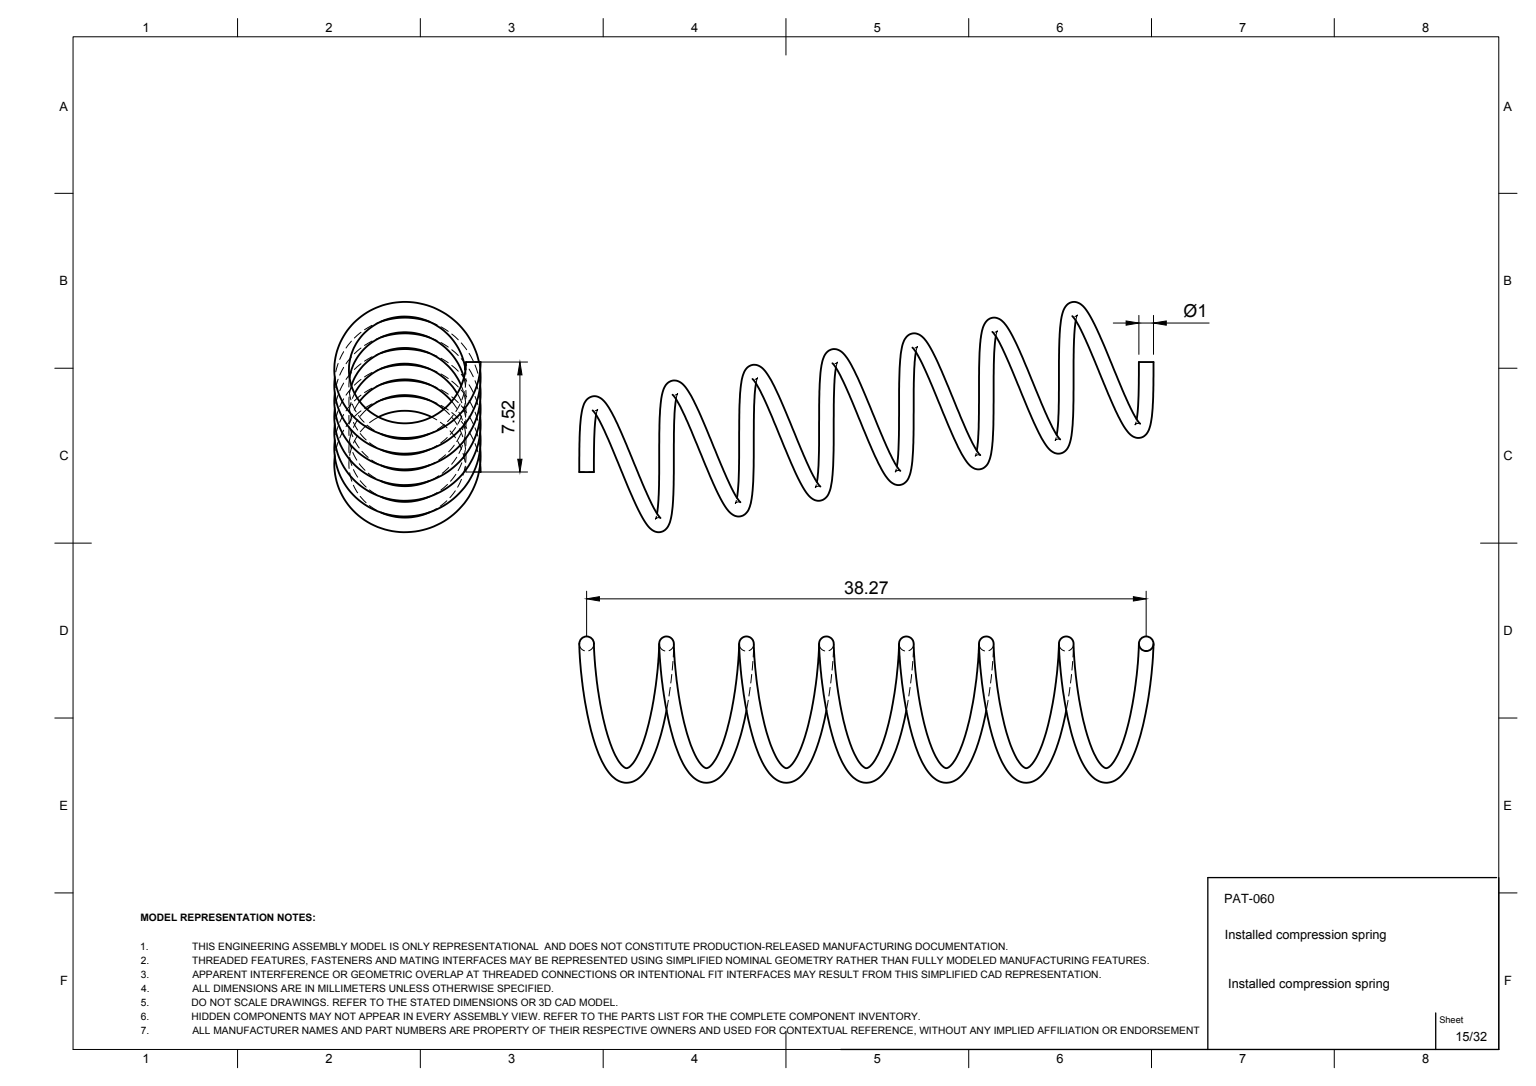
ISO-10303-21;
HEADER;
/* Generated by software containing ST-Developer
 * from STEP Tools, Inc. (www.steptools.com) 
 */

FILE_DESCRIPTION(
/* description */ ('Indexing fixture plate with plunger'),
/* implementation_level */ '2;1');

FILE_NAME(
/* name */ 'Installed compression spring.step',
/* time_stamp */ '2026-10-28T03:23:41-07:00',
/* author */ (''),
/* organization */ (''),
/* preprocessor_version */ 'ST-DEVELOPER v20.2',
/* originating_system */ 'Autodesk Translation Framework v15.17.0.0',
/* authorisation */ '');

FILE_SCHEMA (('AUTOMOTIVE_DESIGN { 1 0 10303 214 3 1 1 }'));
ENDSEC;

DATA;
#10=MECHANICAL_DESIGN_GEOMETRIC_PRESENTATION_REPRESENTATION('',(#327),#10020);
#233=B_SPLINE_SURFACE_WITH_KNOTS('',3,3,((#7454,#7455,#7456,#7457,#7458,
#7459,#7460,#7461,#7462,#7463,#7464,#7465,#7466,#7467,#7468,#7469,#7470,
#7471,#7472,#7473,#7474,#7475,#7476,#7477,#7478,#7479,#7480,#7481,#7482,
#7483,#7484,#7485,#7486,#7487,#7488,#7489,#7490,#7491,#7492,#7493,#7494,
#7495,#7496,#7497,#7498,#7499,#7500,#7501,#7502,#7503,#7504,#7505,#7506,
#7507,#7508,#7509,#7510,#7511,#7512,#7513,#7514,#7515,#7516,#7517,#7518,
#7519,#7520,#7521,#7522,#7523,#7524,#7525,#7526,#7527,#7528,#7529,#7530,
#7531,#7532,#7533,#7534,#7535,#7536,#7537,#7538,#7539,#7540,#7541,#7542,
#7543,#7544,#7545,#7546,#7547,#7548,#7549),(#7550,#7551,#7552,#7553,#7554,
#7555,#7556,#7557,#7558,#7559,#7560,#7561,#7562,#7563,#7564,#7565,#7566,
#7567,#7568,#7569,#7570,#7571,#7572,#7573,#7574,#7575,#7576,#7577,#7578,
#7579,#7580,#7581,#7582,#7583,#7584,#7585,#7586,#7587,#7588,#7589,#7590,
#7591,#7592,#7593,#7594,#7595,#7596,#7597,#7598,#7599,#7600,#7601,#7602,
#7603,#7604,#7605,#7606,#7607,#7608,#7609,#7610,#7611,#7612,#7613,#7614,
#7615,#7616,#7617,#7618,#7619,#7620,#7621,#7622,#7623,#7624,#7625,#7626,
#7627,#7628,#7629,#7630,#7631,#7632,#7633,#7634,#7635,#7636,#7637,#7638,
#7639,#7640,#7641,#7642,#7643,#7644,#7645),(#7646,#7647,#7648,#7649,#7650,
#7651,#7652,#7653,#7654,#7655,#7656,#7657,#7658,#7659,#7660,#7661,#7662,
#7663,#7664,#7665,#7666,#7667,#7668,#7669,#7670,#7671,#7672,#7673,#7674,
#7675,#7676,#7677,#7678,#7679,#7680,#7681,#7682,#7683,#7684,#7685,#7686,
#7687,#7688,#7689,#7690,#7691,#7692,#7693,#7694,#7695,#7696,#7697,#7698,
#7699,#7700,#7701,#7702,#7703,#7704,#7705,#7706,#7707,#7708,#7709,#7710,
#7711,#7712,#7713,#7714,#7715,#7716,#7717,#7718,#7719,#7720,#7721,#7722,
#7723,#7724,#7725,#7726,#7727,#7728,#7729,#7730,#7731,#7732,#7733,#7734,
#7735,#7736,#7737,#7738,#7739,#7740,#7741),(#7742,#7743,#7744,#7745,#7746,
#7747,#7748,#7749,#7750,#7751,#7752,#7753,#7754,#7755,#7756,#7757,#7758,
#7759,#7760,#7761,#7762,#7763,#7764,#7765,#7766,#7767,#7768,#7769,#7770,
#7771,#7772,#7773,#7774,#7775,#7776,#7777,#7778,#7779,#7780,#7781,#7782,
#7783,#7784,#7785,#7786,#7787,#7788,#7789,#7790,#7791,#7792,#7793,#7794,
#7795,#7796,#7797,#7798,#7799,#7800,#7801,#7802,#7803,#7804,#7805,#7806,
#7807,#7808,#7809,#7810,#7811,#7812,#7813,#7814,#7815,#7816,#7817,#7818,
#7819,#7820,#7821,#7822,#7823,#7824,#7825,#7826,#7827,#7828,#7829,#7830,
#7831,#7832,#7833,#7834,#7835,#7836,#7837),(#7838,#7839,#7840,#7841,#7842,
#7843,#7844,#7845,#7846,#7847,#7848,#7849,#7850,#7851,#7852,#7853,#7854,
#7855,#7856,#7857,#7858,#7859,#7860,#7861,#7862,#7863,#7864,#7865,#7866,
#7867,#7868,#7869,#7870,#7871,#7872,#7873,#7874,#7875,#7876,#7877,#7878,
#7879,#7880,#7881,#7882,#7883,#7884,#7885,#7886,#7887,#7888,#7889,#7890,
#7891,#7892,#7893,#7894,#7895,#7896,#7897,#7898,#7899,#7900,#7901,#7902,
#7903,#7904,#7905,#7906,#7907,#7908,#7909,#7910,#7911,#7912,#7913,#7914,
#7915,#7916,#7917,#7918,#7919,#7920,#7921,#7922,#7923,#7924,#7925,#7926,
#7927,#7928,#7929,#7930,#7931,#7932,#7933),(#7934,#7935,#7936,#7937,#7938,
#7939,#7940,#7941,#7942,#7943,#7944,#7945,#7946,#7947,#7948,#7949,#7950,
#7951,#7952,#7953,#7954,#7955,#7956,#7957,#7958,#7959,#7960,#7961,#7962,
#7963,#7964,#7965,#7966,#7967,#7968,#7969,#7970,#7971,#7972,#7973,#7974,
#7975,#7976,#7977,#7978,#7979,#7980,#7981,#7982,#7983,#7984,#7985,#7986,
#7987,#7988,#7989,#7990,#7991,#7992,#7993,#7994,#7995,#7996,#7997,#7998,
#7999,#8000,#8001,#8002,#8003,#8004,#8005,#8006,#8007,#8008,#8009,#8010,
#8011,#8012,#8013,#8014,#8015,#8016,#8017,#8018,#8019,#8020,#8021,#8022,
#8023,#8024,#8025,#8026,#8027,#8028,#8029),(#8030,#8031,#8032,#8033,#8034,
#8035,#8036,#8037,#8038,#8039,#8040,#8041,#8042,#8043,#8044,#8045,#8046,
#8047,#8048,#8049,#8050,#8051,#8052,#8053,#8054,#8055,#8056,#8057,#8058,
#8059,#8060,#8061,#8062,#8063,#8064,#8065,#8066,#8067,#8068,#8069,#8070,
#8071,#8072,#8073,#8074,#8075,#8076,#8077,#8078,#8079,#8080,#8081,#8082,
#8083,#8084,#8085,#8086,#8087,#8088,#8089,#8090,#8091,#8092,#8093,#8094,
#8095,#8096,#8097,#8098,#8099,#8100,#8101,#8102,#8103,#8104,#8105,#8106,
#8107,#8108,#8109,#8110,#8111,#8112,#8113,#8114,#8115,#8116,#8117,#8118,
#8119,#8120,#8121,#8122,#8123,#8124,#8125),(#8126,#8127,#8128,#8129,#8130,
#8131,#8132,#8133,#8134,#8135,#8136,#8137,#8138,#8139,#8140,#8141,#8142,
#8143,#8144,#8145,#8146,#8147,#8148,#8149,#8150,#8151,#8152,#8153,#8154,
#8155,#8156,#8157,#8158,#8159,#8160,#8161,#8162,#8163,#8164,#8165,#8166,
#8167,#8168,#8169,#8170,#8171,#8172,#8173,#8174,#8175,#8176,#8177,#8178,
#8179,#8180,#8181,#8182,#8183,#8184,#8185,#8186,#8187,#8188,#8189,#8190,
#8191,#8192,#8193,#8194,#8195,#8196,#8197,#8198,#8199,#8200,#8201,#8202,
#8203,#8204,#8205,#8206,#8207,#8208,#8209,#8210,#8211,#8212,#8213,#8214,
#8215,#8216,#8217,#8218,#8219,#8220,#8221),(#8222,#8223,#8224,#8225,#8226,
#8227,#8228,#8229,#8230,#8231,#8232,#8233,#8234,#8235,#8236,#8237,#8238,
#8239,#8240,#8241,#8242,#8243,#8244,#8245,#8246,#8247,#8248,#8249,#8250,
#8251,#8252,#8253,#8254,#8255,#8256,#8257,#8258,#8259,#8260,#8261,#8262,
#8263,#8264,#8265,#8266,#8267,#8268,#8269,#8270,#8271,#8272,#8273,#8274,
#8275,#8276,#8277,#8278,#8279,#8280,#8281,#8282,#8283,#8284,#8285,#8286,
#8287,#8288,#8289,#8290,#8291,#8292,#8293,#8294,#8295,#8296,#8297,#8298,
#8299,#8300,#8301,#8302,#8303,#8304,#8305,#8306,#8307,#8308,#8309,#8310,
#8311,#8312,#8313,#8314,#8315,#8316,#8317),(#8318,#8319,#8320,#8321,#8322,
#8323,#8324,#8325,#8326,#8327,#8328,#8329,#8330,#8331,#8332,#8333,#8334,
#8335,#8336,#8337,#8338,#8339,#8340,#8341,#8342,#8343,#8344,#8345,#8346,
#8347,#8348,#8349,#8350,#8351,#8352,#8353,#8354,#8355,#8356,#8357,#8358,
#8359,#8360,#8361,#8362,#8363,#8364,#8365,#8366,#8367,#8368,#8369,#8370,
#8371,#8372,#8373,#8374,#8375,#8376,#8377,#8378,#8379,#8380,#8381,#8382,
#8383,#8384,#8385,#8386,#8387,#8388,#8389,#8390,#8391,#8392,#8393,#8394,
#8395,#8396,#8397,#8398,#8399,#8400,#8401,#8402,#8403,#8404,#8405,#8406,
#8407,#8408,#8409,#8410,#8411,#8412,#8413)),.UNSPECIFIED.,.T.,.F.,.F.,(4,
1,1,1,1,1,1,4),(4,1,1,1,1,1,1,1,1,1,1,1,1,1,1,1,1,1,1,1,1,1,1,1,1,1,1,1,
1,1,1,1,1,1,1,1,1,1,1,1,1,1,1,1,1,1,1,1,1,1,1,1,1,1,1,1,1,1,1,1,1,1,1,1,
1,1,1,1,1,1,1,1,1,1,1,1,1,1,1,1,1,1,1,1,1,1,1,1,1,1,1,1,1,4),(-3.14159265358979,
-2.24399475256414,-1.34639685153848,-0.448798950512828,0.448798950512828,
1.34639685153848,2.24399475256414,3.14159265358979),(0.,0.00892857142857143,
0.0178571428571429,0.0267857142857143,0.0357142857142857,0.0446428571428571,
0.0535714285714286,0.0625,0.0714285714285714,0.0803571428571428,0.0892857142857143,
0.107142857142857,0.125,0.133928571428571,0.142857142857143,0.158730158730159,
0.174603174603175,0.19047619047619,0.202380952380952,0.214285714285714,
0.226190476190476,0.238095238095238,0.25,0.261904761904762,0.273809523809524,
0.285714285714286,0.297619047619048,0.30952380952381,0.321428571428571,
0.333333333333333,0.345238095238095,0.357142857142857,0.369047619047619,
0.375,0.380952380952381,0.392857142857143,0.404761904761905,0.416666666666667,
0.428571428571429,0.4375,0.446428571428571,0.455357142857143,0.464285714285714,
0.476190476190476,0.488095238095238,0.5,0.508928571428571,0.517857142857143,
0.535714285714286,0.553571428571429,0.571428571428571,0.580357142857143,
0.589285714285714,0.598214285714286,0.607142857142857,0.616071428571429,
0.625,0.633928571428571,0.642857142857143,0.654761904761905,0.666666666666667,
0.678571428571428,0.6875,0.696428571428571,0.705357142857143,0.714285714285714,
0.726190476190476,0.738095238095238,0.75,0.761904761904762,0.773809523809524,
0.785714285714286,0.797619047619047,0.809523809523809,0.821428571428571,
0.833333333333333,0.845238095238095,0.857142857142857,0.866071428571429,
0.875,0.883928571428571,0.892857142857143,0.901785714285714,0.910714285714286,
0.919642857142857,0.928571428571429,0.9375,0.946428571428571,0.955357142857143,
0.964285714285714,0.973214285714286,0.982142857142857,0.991071428571429,
1.),.UNSPECIFIED.);
#239=B_SPLINE_CURVE_WITH_KNOTS('',3,(#8417,#8418,#8419,#8420,#8421,#8422,
#8423,#8424,#8425,#8426,#8427,#8428,#8429,#8430,#8431,#8432,#8433,#8434,
#8435,#8436,#8437,#8438,#8439,#8440,#8441,#8442,#8443,#8444,#8445,#8446,
#8447,#8448,#8449,#8450,#8451,#8452,#8453,#8454,#8455,#8456,#8457,#8458,
#8459,#8460,#8461,#8462,#8463,#8464,#8465,#8466,#8467,#8468,#8469,#8470,
#8471,#8472,#8473,#8474,#8475,#8476,#8477,#8478,#8479,#8480,#8481,#8482,
#8483,#8484,#8485,#8486,#8487,#8488,#8489,#8490,#8491,#8492,#8493,#8494,
#8495,#8496,#8497,#8498,#8499,#8500,#8501,#8502,#8503,#8504,#8505,#8506,
#8507,#8508,#8509,#8510,#8511,#8512),.UNSPECIFIED.,.F.,.F.,(4,1,1,1,1,1,
1,1,1,1,1,1,1,1,1,1,1,1,1,1,1,1,1,1,1,1,1,1,1,1,1,1,1,1,1,1,1,1,1,1,1,1,
1,1,1,1,1,1,1,1,1,1,1,1,1,1,1,1,1,1,1,1,1,1,1,1,1,1,1,1,1,1,1,1,1,1,1,1,
1,1,1,1,1,1,1,1,1,1,1,1,1,1,1,4),(0.,0.00892857142857143,0.0178571428571429,
0.0267857142857143,0.0357142857142857,0.0446428571428571,0.0535714285714286,
0.0625,0.0714285714285714,0.0803571428571428,0.0892857142857143,0.107142857142857,
0.125,0.133928571428571,0.142857142857143,0.158730158730159,0.174603174603175,
0.19047619047619,0.202380952380952,0.214285714285714,0.226190476190476,
0.238095238095238,0.25,0.261904761904762,0.273809523809524,0.285714285714286,
0.297619047619048,0.30952380952381,0.321428571428571,0.333333333333333,
0.345238095238095,0.357142857142857,0.369047619047619,0.375,0.380952380952381,
0.392857142857143,0.404761904761905,0.416666666666667,0.428571428571429,
0.4375,0.446428571428571,0.455357142857143,0.464285714285714,0.476190476190476,
0.488095238095238,0.5,0.508928571428571,0.517857142857143,0.535714285714286,
0.553571428571429,0.571428571428571,0.580357142857143,0.589285714285714,
0.598214285714286,0.607142857142857,0.616071428571429,0.625,0.633928571428571,
0.642857142857143,0.654761904761905,0.666666666666667,0.678571428571428,
0.6875,0.696428571428571,0.705357142857143,0.714285714285714,0.726190476190476,
0.738095238095238,0.75,0.761904761904762,0.773809523809524,0.785714285714286,
0.797619047619047,0.809523809523809,0.821428571428571,0.833333333333333,
0.845238095238095,0.857142857142857,0.866071428571429,0.875,0.883928571428571,
0.892857142857143,0.901785714285714,0.910714285714286,0.919642857142857,
0.928571428571429,0.9375,0.946428571428571,0.955357142857143,0.964285714285714,
0.973214285714286,0.982142857142857,0.991071428571429,1.),.UNSPECIFIED.);
#273=SHAPE_REPRESENTATION_RELATIONSHIP('SRR','None',#10147,#300);
#300=ADVANCED_BREP_SHAPE_REPRESENTATION('',(#363),#10000);
#327=STYLED_ITEM('',(#10368),#363);
#363=MANIFOLD_SOLID_BREP('Body1',#4581);
#568=PLANE('',#5049);
#569=PLANE('',#5050);
#733=FACE_OUTER_BOUND('',#1060,.T.);
#734=FACE_OUTER_BOUND('',#1061,.T.);
#735=FACE_OUTER_BOUND('',#1062,.T.);
#1060=EDGE_LOOP('',(#3293,#3294,#3295,#3296));
#1061=EDGE_LOOP('',(#3297));
#1062=EDGE_LOOP('',(#3298));
#1896=CIRCLE('',#5047,0.05);
#1897=CIRCLE('',#5048,0.05);
#2212=VERTEX_POINT('',#8414);
#2213=VERTEX_POINT('',#8416);
#2626=EDGE_CURVE('',#2212,#2212,#1896,.T.);
#2627=EDGE_CURVE('',#2212,#2213,#239,.T.);
#2628=EDGE_CURVE('',#2213,#2213,#1897,.T.);
#3293=ORIENTED_EDGE('',*,*,#2626,.T.);
#3294=ORIENTED_EDGE('',*,*,#2627,.T.);
#3295=ORIENTED_EDGE('',*,*,#2628,.F.);
#3296=ORIENTED_EDGE('',*,*,#2627,.F.);
#3297=ORIENTED_EDGE('',*,*,#2628,.T.);
#3298=ORIENTED_EDGE('',*,*,#2626,.F.);
#4348=ADVANCED_FACE('',(#733),#233,.T.);
#4349=ADVANCED_FACE('',(#734),#568,.T.);
#4350=ADVANCED_FACE('',(#735),#569,.F.);
#4581=CLOSED_SHELL('',(#4348,#4349,#4350));
#5046=AXIS2_PLACEMENT_3D('',#7453,#5897,#5898);
#5047=AXIS2_PLACEMENT_3D('',#8415,#5899,#5900);
#5048=AXIS2_PLACEMENT_3D('',#8513,#5901,#5902);
#5049=AXIS2_PLACEMENT_3D('',#8514,#5903,#5904);
#5050=AXIS2_PLACEMENT_3D('',#8515,#5905,#5906);
#5897=DIRECTION('axis',(0.,0.,1.));
#5898=DIRECTION('refdir',(1.,0.,0.));
#5899=DIRECTION('center_axis',(-0.000132267085706657,0.981242764302753,
0.192776087751852));
#5900=DIRECTION('ref_axis',(2.59853443172113E-5,-0.192776086000499,0.981242773217255));
#5901=DIRECTION('center_axis',(0.000132265595059966,0.981242764048193,0.192776089048605));
#5902=DIRECTION('ref_axis',(-0.796598144949105,0.116638308439033,-0.593149981428075));
#5903=DIRECTION('center_axis',(0.000132265595059966,0.981242764048193,0.192776089048605));
#5904=DIRECTION('ref_axis',(-0.796598144949105,0.116638308439033,-0.593149981428075));
#5905=DIRECTION('center_axis',(-0.000132267085706657,0.981242764302753,
0.192776087751852));
#5906=DIRECTION('ref_axis',(2.59853443172113E-5,-0.192776086000499,0.981242773217256));
#7453=CARTESIAN_POINT('',(0.,0.,0.));
#7454=CARTESIAN_POINT('Ctrl Pts',(7.64999870073278,0.00963880430002493,
0.500937861339137));
#7455=CARTESIAN_POINT('Ctrl Pts',(7.64999072283273,0.0688240253405825,0.512565458280486));
#7456=CARTESIAN_POINT('Ctrl Pts',(7.62651906829351,0.186933280416436,0.535860737255745));
#7457=CARTESIAN_POINT('Ctrl Pts',(7.52538952050926,0.338721501716328,0.571111621876026));
#7458=CARTESIAN_POINT('Ctrl Pts',(7.37261016576107,0.440828782725881,0.606632113855559));
#7459=CARTESIAN_POINT('Ctrl Pts',(7.19098801918939,0.477160089388571,0.642432691908446));
#7460=CARTESIAN_POINT('Ctrl Pts',(7.00794887133667,0.440792445335284,0.678501299793522));
#7461=CARTESIAN_POINT('Ctrl Pts',(6.85151949944076,0.336499171833787,0.714833893830788));
#7462=CARTESIAN_POINT('Ctrl Pts',(6.74635289761356,0.179164878106423,0.751420068859459));
#7463=CARTESIAN_POINT('Ctrl Pts',(6.7088855037237,-0.00779582609077112,
0.78825059826266));
#7464=CARTESIAN_POINT('Ctrl Pts',(6.74651391108833,-0.195622387289353,0.825313313466632));
#7465=CARTESIAN_POINT('Ctrl Pts',(6.88851119015049,-0.410310488976418,0.875022999496246));
#7466=CARTESIAN_POINT('Ctrl Pts',(7.20522985356176,-0.542753193552164,0.937673401670968));
#7467=CARTESIAN_POINT('Ctrl Pts',(7.52560124560565,-0.410308950963103,1.00090311405878));
#7468=CARTESIAN_POINT('Ctrl Pts',(7.67086762315913,-0.190619832396083,1.0517623380234));
#7469=CARTESIAN_POINT('Ctrl Pts',(7.72038428103372,0.053554354178951,1.09994516441643));
#7470=CARTESIAN_POINT('Ctrl Pts',(7.61346157902179,0.349425527858921,1.15825605943124));
#7471=CARTESIAN_POINT('Ctrl Pts',(7.293147036645,0.533923363778534,1.22671892603372));
#7472=CARTESIAN_POINT('Ctrl Pts',(6.9598052915743,0.475238618295502,1.28954716027338));
#7473=CARTESIAN_POINT('Ctrl Pts',(6.74803078150055,0.262318163018047,1.34663189357301));
#7474=CARTESIAN_POINT('Ctrl Pts',(6.67830810206772,0.0023988076890563,1.3979329504908));
#7475=CARTESIAN_POINT('Ctrl Pts',(6.74786353789082,-0.257385664114871,1.44910892564238));
#7476=CARTESIAN_POINT('Ctrl Pts',(6.93745136291826,-0.446625861944449,1.50011118169226));
#7477=CARTESIAN_POINT('Ctrl Pts',(7.19511270617401,-0.515530236866011,1.55089291586215));
#7478=CARTESIAN_POINT('Ctrl Pts',(7.45136837615866,-0.446648689171563,1.60140954707133));
#7479=CARTESIAN_POINT('Ctrl Pts',(7.63768442718454,-0.260018056286165,1.65161922462518));
#7480=CARTESIAN_POINT('Ctrl Pts',(7.70523033687804,-0.0069714683683192,
1.70148323387221));
#7481=CARTESIAN_POINT('Ctrl Pts',(7.63769895751989,0.244003419049979,1.75096640161628));
#7482=CARTESIAN_POINT('Ctrl Pts',(7.45523859330254,0.426040600914326,1.80003745460796));
#7483=CARTESIAN_POINT('Ctrl Pts',(7.20843773134158,0.491855409637758,1.84866933496872));
#7484=CARTESIAN_POINT('Ctrl Pts',(6.96411419073211,0.426044527968114,1.89683949153479));
#7485=CARTESIAN_POINT('Ctrl Pts',(6.7872702247347,0.248717255937941,1.94453007704133));
#7486=CARTESIAN_POINT('Ctrl Pts',(6.72333142706999,0.00910740273079913,
1.99172820696913));
#7487=CARTESIAN_POINT('Ctrl Pts',(6.77669190792476,-0.188112629887261,2.03064296753181));
#7488=CARTESIAN_POINT('Ctrl Pts',(6.87311288530633,-0.313353108724919,2.06152326719269));
#7489=CARTESIAN_POINT('Ctrl Pts',(6.9977575234091,-0.409174440391491,2.0922362142172));
#7490=CARTESIAN_POINT('Ctrl Pts',(7.19095586866206,-0.460713817161615,2.13031448846159));
#7491=CARTESIAN_POINT('Ctrl Pts',(7.42021304552618,-0.399036009194613,2.17551521533059));
#7492=CARTESIAN_POINT('Ctrl Pts',(7.58607675038944,-0.232652998639623,2.22023530187249));
#7493=CARTESIAN_POINT('Ctrl Pts',(7.64084113722653,-0.0267711157317457,
2.2608041635776));
#7494=CARTESIAN_POINT('Ctrl Pts',(7.60365245023964,0.158696418911201,2.2973634945418));
#7495=CARTESIAN_POINT('Ctrl Pts',(7.50973838584388,0.299219822341778,2.33003006433835));
#7496=CARTESIAN_POINT('Ctrl Pts',(7.37007100234203,0.392281683236922,2.36247215334549));
#7497=CARTESIAN_POINT('Ctrl Pts',(7.18832364110351,0.428509871500047,2.39828479951764));
#7498=CARTESIAN_POINT('Ctrl Pts',(6.98993152312495,0.375130255900093,2.43739940337039));
#7499=CARTESIAN_POINT('Ctrl Pts',(6.83283942785452,0.217642962930976,2.47976008769737));
#7500=CARTESIAN_POINT('Ctrl Pts',(6.7805179762894,0.0217759129571612,2.51834494637949));
#7501=CARTESIAN_POINT('Ctrl Pts',(6.81611962546049,-0.155110783437508,2.55325894844757));
#7502=CARTESIAN_POINT('Ctrl Pts',(6.93559514558806,-0.335467183812974,2.59501419582854));
#7503=CARTESIAN_POINT('Ctrl Pts',(7.19838636703693,-0.444497554803198,2.64699296075227));
#7504=CARTESIAN_POINT('Ctrl Pts',(7.51396784981042,-0.313675439428632,2.70919005501935));
#7505=CARTESIAN_POINT('Ctrl Pts',(7.62212313812957,-0.0514208051434247,
2.76101600110827));
#7506=CARTESIAN_POINT('Ctrl Pts',(7.57941022831611,0.159498854704775,2.80255943176652));
#7507=CARTESIAN_POINT('Ctrl Pts',(7.49002790476542,0.293811387305209,2.83377939972915));
#7508=CARTESIAN_POINT('Ctrl Pts',(7.3552499441484,0.383795703607156,2.86508254302445));
#7509=CARTESIAN_POINT('Ctrl Pts',(7.19595280633545,0.41560735445773,2.89648910888395));
#7510=CARTESIAN_POINT('Ctrl Pts',(7.03593949389396,0.383792650446306,2.92801879141503));
#7511=CARTESIAN_POINT('Ctrl Pts',(6.89961651509014,0.292876470296345,2.95969053299985));
#7512=CARTESIAN_POINT('Ctrl Pts',(6.8081238548802,0.155952445855146,2.99152250722056));
#7513=CARTESIAN_POINT('Ctrl Pts',(6.7719951154116,-0.0244720795860329,3.02708849903104));
#7514=CARTESIAN_POINT('Ctrl Pts',(6.82508694038131,-0.224423780156864,3.0664872528009));
#7515=CARTESIAN_POINT('Ctrl Pts',(6.9861130399098,-0.385566648672682,3.1098474493302));
#7516=CARTESIAN_POINT('Ctrl Pts',(7.18949761386412,-0.440411898981026,3.14997109794484));
#7517=CARTESIAN_POINT('Ctrl Pts',(7.37626527013998,-0.403213775048244,3.18676673081186));
#7518=CARTESIAN_POINT('Ctrl Pts',(7.51993103796524,-0.30750405465344,3.2201390303787));
#7519=CARTESIAN_POINT('Ctrl Pts',(7.61665044076158,-0.16281791922389,3.25377599756719));
#7520=CARTESIAN_POINT('Ctrl Pts',(7.65498225700094,0.0283123086785322,3.29145196922942));
#7521=CARTESIAN_POINT('Ctrl Pts',(7.59852316170633,0.240631420079613,3.3332902111484));
#7522=CARTESIAN_POINT('Ctrl Pts',(7.42736589163809,0.412328652603764,3.37943210760514));
#7523=CARTESIAN_POINT('Ctrl Pts',(7.19081184831391,0.475941162716025,3.42607713455886));
#7524=CARTESIAN_POINT('Ctrl Pts',(6.95151342469985,0.412204069493947,3.47322302929114));
#7525=CARTESIAN_POINT('Ctrl Pts',(6.77437422620912,0.235528496642651,3.52086247665056));
#7526=CARTESIAN_POINT('Ctrl Pts',(6.70856719057301,-0.00853695568196444,
3.56898306053165));
#7527=CARTESIAN_POINT('Ctrl Pts',(6.77444746404088,-0.255049338492359,3.61756749823055));
#7528=CARTESIAN_POINT('Ctrl Pts',(6.9562898685306,-0.437346140614658,3.66659366870206));
#7529=CARTESIAN_POINT('Ctrl Pts',(7.20705837195632,-0.504822359013845,3.71603499825878));
#7530=CARTESIAN_POINT('Ctrl Pts',(7.45987118758895,-0.437340247483335,3.76586064283255));
#7531=CARTESIAN_POINT('Ctrl Pts',(7.64643847266503,-0.251145802482984,3.81603581337119));
#7532=CARTESIAN_POINT('Ctrl Pts',(7.70939130979041,-0.0164226811455054,
3.86231497498143));
#7533=CARTESIAN_POINT('Ctrl Pts',(7.66665300702434,0.198091300428752,3.90458351454994));
#7534=CARTESIAN_POINT('Ctrl Pts',(7.55703831361006,0.362363180751678,3.94275824199772));
#7535=CARTESIAN_POINT('Ctrl Pts',(7.39231161872226,0.472405147713809,3.98104671473859));
#7536=CARTESIAN_POINT('Ctrl Pts',(7.19757748614764,0.511253819560404,4.01942894411337));
#7537=CARTESIAN_POINT('Ctrl Pts',(7.00243742159468,0.472394913482402,4.05788442705078));
#7538=CARTESIAN_POINT('Ctrl Pts',(6.83675859423202,0.361776141956741,4.09639221672569));
#7539=CARTESIAN_POINT('Ctrl Pts',(6.72593678453896,0.195994806221917,4.13493108529455));
#7540=CARTESIAN_POINT('Ctrl Pts',(6.6870196897812,0.000372767277272366,
4.17347960299015));
#7541=CARTESIAN_POINT('Ctrl Pts',(6.72599808190112,-0.19515902350661,4.21201632288769));
#7542=CARTESIAN_POINT('Ctrl Pts',(6.83662574734572,-0.360840864201945,4.25051978478148));
#7543=CARTESIAN_POINT('Ctrl Pts',(7.00208504736442,-0.47127212461887,4.28896891774833));
#7544=CARTESIAN_POINT('Ctrl Pts',(7.19679737636779,-0.510060779189973,4.32734248506513));
#7545=CARTESIAN_POINT('Ctrl Pts',(7.39100313831524,-0.471299286801184,4.36562087591661));
#7546=CARTESIAN_POINT('Ctrl Pts',(7.5551719819179,-0.361667391724164,4.40378216412631));
#7547=CARTESIAN_POINT('Ctrl Pts',(7.66435033350436,-0.197951056928272,4.44181269280615));
#7548=CARTESIAN_POINT('Ctrl Pts',(7.68982126235038,-0.0699660743691742,
4.46705762798012));
#7549=CARTESIAN_POINT('Ctrl Pts',(7.68982990724746,-0.00583191542195246,
4.4796574990714));
#7550=CARTESIAN_POINT('Ctrl Pts',(7.6350387358516,0.00963678776443446,0.500937861339137));
#7551=CARTESIAN_POINT('Ctrl Pts',(7.63503101014841,0.0669510493656743,0.512197887426284));
#7552=CARTESIAN_POINT('Ctrl Pts',(7.61231574924475,0.1812935300152,0.5347473807854));
#7553=CARTESIAN_POINT('Ctrl Pts',(7.51437536109004,0.328330400226009,0.568888525111363));
#7554=CARTESIAN_POINT('Ctrl Pts',(7.36630661624771,0.427307066398246,0.603312533918598));
#7555=CARTESIAN_POINT('Ctrl Pts',(7.19013369937419,0.462570873330364,0.638036216400197));
#7556=CARTESIAN_POINT('Ctrl Pts',(7.01240713420346,0.42727728453773,0.673054009319043));
#7557=CARTESIAN_POINT('Ctrl Pts',(6.86033508130397,0.325921179563573,0.70836726659389));
#7558=CARTESIAN_POINT('Ctrl Pts',(6.7579611971146,0.172802978923407,0.74397206566071));
#7559=CARTESIAN_POINT('Ctrl Pts',(6.7214123199082,-0.00940771975300016,
0.779864408487187));
#7560=CARTESIAN_POINT('Ctrl Pts',(6.7581198571664,-0.192756797259193,0.816037450325855));
#7561=CARTESIAN_POINT('Ctrl Pts',(6.89690232809005,-0.402672103199899,0.86463407058812));
#7562=CARTESIAN_POINT('Ctrl Pts',(7.20725605051053,-0.532709504267443,0.926031233812609));
#7563=CARTESIAN_POINT('Ctrl Pts',(7.52258283785506,-0.402635707082477,0.988237247131344));
#7564=CARTESIAN_POINT('Ctrl Pts',(7.66601723416036,-0.185829339954806,1.0384238006937));
#7565=CARTESIAN_POINT('Ctrl Pts',(7.71503355357269,0.0556422780873975,1.08607199043942));
#7566=CARTESIAN_POINT('Ctrl Pts',(7.60918637088204,0.349162880547258,1.14388762640479));
#7567=CARTESIAN_POINT('Ctrl Pts',(7.2903515128854,0.533103613911741,1.21204744313397));
#7568=CARTESIAN_POINT('Ctrl Pts',(6.95707366748621,0.474656316327783,1.27485358832891));
#7569=CARTESIAN_POINT('Ctrl Pts',(6.74456178112433,0.261169820551568,1.33209897131474));
#7570=CARTESIAN_POINT('Ctrl Pts',(6.67433527221315,-0.000269397014741131,
1.38369681229794));
#7571=CARTESIAN_POINT('Ctrl Pts',(6.74440593081803,-0.262373809003338,1.43532105174058));
#7572=CARTESIAN_POINT('Ctrl Pts',(6.93612728066397,-0.453872081669123,1.48690459984704));
#7573=CARTESIAN_POINT('Ctrl Pts',(7.19745122001508,-0.523848922372219,1.53840681076736));
#7574=CARTESIAN_POINT('Ctrl Pts',(7.45805997886714,-0.453883269663763,1.58977025772498));
#7575=CARTESIAN_POINT('Ctrl Pts',(7.64803983262086,-0.263693101035238,1.64094678753314));
#7576=CARTESIAN_POINT('Ctrl Pts',(7.71711952609534,-0.00517849878257243,
1.69188667453881));
#7577=CARTESIAN_POINT('Ctrl Pts',(7.64804216604535,0.251791239903175,1.74254418096352));
#7578=CARTESIAN_POINT('Ctrl Pts',(7.46092188629594,0.438558185201571,1.79287579243366));
#7579=CARTESIAN_POINT('Ctrl Pts',(7.20735063505956,0.506228936588262,1.8428415890961));
#7580=CARTESIAN_POINT('Ctrl Pts',(6.95593925559357,0.438549903941295,1.89240539488024));
#7581=CARTESIAN_POINT('Ctrl Pts',(6.77373440484268,0.255889979988123,1.94153491121713));
#7582=CARTESIAN_POINT('Ctrl Pts',(6.70778531151454,0.00882356266419227,
1.99020293693628));
#7583=CARTESIAN_POINT('Ctrl Pts',(6.76283355713105,-0.194668074958629,2.0303550609426));
#7584=CARTESIAN_POINT('Ctrl Pts',(6.86234426891409,-0.323919294450078,2.06222522567205));
#7585=CARTESIAN_POINT('Ctrl Pts',(6.99099241075521,-0.4228168735756,2.09392553998431));
#7586=CARTESIAN_POINT('Ctrl Pts',(7.19040501251761,-0.476002229606067,2.1332315590035));
#7587=CARTESIAN_POINT('Ctrl Pts',(7.42694509743174,-0.412343436770496,2.17987197648186));
#7588=CARTESIAN_POINT('Ctrl Pts',(7.59795477669367,-0.24075224108209,2.22599099832676));
#7589=CARTESIAN_POINT('Ctrl Pts',(7.65432879696381,-0.0286540038200118,
2.26778999749925));
#7590=CARTESIAN_POINT('Ctrl Pts',(7.61604593360169,0.162166641626849,2.30540718503675));
#7591=CARTESIAN_POINT('Ctrl Pts',(7.51950918270181,0.306566623965249,2.33898210158965));
#7592=CARTESIAN_POINT('Ctrl Pts',(7.37615986978507,0.402052531958415,2.3722797613854));
#7593=CARTESIAN_POINT('Ctrl Pts',(7.18991757189564,0.439140491267482,2.40898011568004));
#7594=CARTESIAN_POINT('Ctrl Pts',(6.98704945595601,0.384483438050293,2.44898977868643));
#7595=CARTESIAN_POINT('Ctrl Pts',(6.82687936658702,0.223795186966439,2.49220010365028));
#7596=CARTESIAN_POINT('Ctrl Pts',(6.77374406457618,0.0245525470923147,2.53145813471135));
#7597=CARTESIAN_POINT('Ctrl Pts',(6.80989272676198,-0.154854651698435,2.56687895662991));
#7598=CARTESIAN_POINT('Ctrl Pts',(6.93084711889443,-0.337336060775077,2.60913936898076));
#7599=CARTESIAN_POINT('Ctrl Pts',(7.19586714485277,-0.446979863060233,2.66154817199395));
#7600=CARTESIAN_POINT('Ctrl Pts',(7.51214995264661,-0.315456586630328,2.72392487242511));
#7601=CARTESIAN_POINT('Ctrl Pts',(7.61973089828985,-0.0538169044635309,
2.77562308796219));
#7602=CARTESIAN_POINT('Ctrl Pts',(7.57725516276559,0.155639272831775,2.81688936140585));
#7603=CARTESIAN_POINT('Ctrl Pts',(7.48867898425771,0.288669487348,2.84782028505493));
#7604=CARTESIAN_POINT('Ctrl Pts',(7.35549434227958,0.377544841875494,2.8787535369846));
#7605=CARTESIAN_POINT('Ctrl Pts',(7.19848583194038,0.408858679622143,2.90971124099487));
#7606=CARTESIAN_POINT('Ctrl Pts',(7.0411630337891,0.37754703996107,2.94071683444724));
#7607=CARTESIAN_POINT('Ctrl Pts',(6.90744882895457,0.288327999365551,2.97179002108998));
#7608=CARTESIAN_POINT('Ctrl Pts',(6.8179071425464,0.154275853325778,3.00295604846018));
#7609=CARTESIAN_POINT('Ctrl Pts',(6.78264236297597,-0.0220015791954167,
3.03770458582966));
#7610=CARTESIAN_POINT('Ctrl Pts',(6.8344572243931,-0.216935347146573,3.07612357321105));
#7611=CARTESIAN_POINT('Ctrl Pts',(6.99115063676539,-0.373674687144112,3.11831302609281));
#7612=CARTESIAN_POINT('Ctrl Pts',(7.18868631032597,-0.426903740536407,3.15728375484868));
#7613=CARTESIAN_POINT('Ctrl Pts',(7.36984365698281,-0.390811492032386,3.19297776573814));
#7614=CARTESIAN_POINT('Ctrl Pts',(7.50907371772657,-0.298044602028427,3.22532144483156));
#7615=CARTESIAN_POINT('Ctrl Pts',(7.60274490909148,-0.15791000624285,3.2579014410467));
#7616=CARTESIAN_POINT('Ctrl Pts',(7.63984896443366,0.0271238759470453,3.2943750240253));
#7617=CARTESIAN_POINT('Ctrl Pts',(7.58520989641712,0.232609561821433,3.33486742258247));
#7618=CARTESIAN_POINT('Ctrl Pts',(7.41956867650539,0.398792804467796,3.37952311993261));
#7619=CARTESIAN_POINT('Ctrl Pts',(7.1905457231359,0.460399855551445,3.42468394189214));
#7620=CARTESIAN_POINT('Ctrl Pts',(6.95869704927801,0.398681696943234,3.47035666953234));
#7621=CARTESIAN_POINT('Ctrl Pts',(6.78688141707536,0.227371623889039,3.51655404942707));
#7622=CARTESIAN_POINT('Ctrl Pts',(6.7229312949975,-0.00960578475399217,
3.5632735819084));
#7623=CARTESIAN_POINT('Ctrl Pts',(6.78694999671625,-0.249365465366649,3.61052175321115));
#7624=CARTESIAN_POINT('Ctrl Pts',(6.96406181917366,-0.427017015476016,3.65827815384324));
#7625=CARTESIAN_POINT('Ctrl Pts',(7.20884449734192,-0.492960246040882,3.70653567209578));
#7626=CARTESIAN_POINT('Ctrl Pts',(7.45620532585719,-0.427018438033829,3.75527364860311));
#7627=CARTESIAN_POINT('Ctrl Pts',(7.63922818507954,-0.244485987870997,3.80447044259358));
#7628=CARTESIAN_POINT('Ctrl Pts',(7.70120240491438,-0.0137441258516156,
3.84995779136607));
#7629=CARTESIAN_POINT('Ctrl Pts',(7.65913006311212,0.197656069537059,3.89160533681384));
#7630=CARTESIAN_POINT('Ctrl Pts',(7.55093165022181,0.359884525576526,3.9292907213808));
#7631=CARTESIAN_POINT('Ctrl Pts',(7.38795046396419,0.468807636689479,3.96717529387949));
#7632=CARTESIAN_POINT('Ctrl Pts',(7.19485944556467,0.507376335556598,4.00522949186857));
#7633=CARTESIAN_POINT('Ctrl Pts',(7.00092895437896,0.468801673803832,4.04343882565719));
#7634=CARTESIAN_POINT('Ctrl Pts',(6.83589776048967,0.358671322852951,4.08178585172935));
#7635=CARTESIAN_POINT('Ctrl Pts',(6.72525082625392,0.193231928470719,4.12024424860606));
#7636=CARTESIAN_POINT('Ctrl Pts',(6.68627533701788,-0.00244208003353348,
4.15880023983475));
#7637=CARTESIAN_POINT('Ctrl Pts',(6.72531069708358,-0.198468266862919,4.19742754656923));
#7638=CARTESIAN_POINT('Ctrl Pts',(6.83641060841933,-0.36494553097655,4.23610417128916));
#7639=CARTESIAN_POINT('Ctrl Pts',(7.00297752232982,-0.476160108331975,4.27480979854181));
#7640=CARTESIAN_POINT('Ctrl Pts',(7.19941745683392,-0.515336210269313,4.313521430379));
#7641=CARTESIAN_POINT('Ctrl Pts',(7.39577334638842,-0.476178009162295,4.35221655573581));
#7642=CARTESIAN_POINT('Ctrl Pts',(7.56210403701843,-0.365136489373791,4.39087303722902));
#7643=CARTESIAN_POINT('Ctrl Pts',(7.6729482105615,-0.198970065641914,4.42946934287203));
#7644=CARTESIAN_POINT('Ctrl Pts',(7.69886454791239,-0.0687900400044386,
4.45514378820058));
#7645=CARTESIAN_POINT('Ctrl Pts',(7.69887334379488,-0.003535760932353,4.46796371938795));
#7646=CARTESIAN_POINT('Ctrl Pts',(7.60521013505817,0.00687058616980481,
0.514997540570331));
#7647=CARTESIAN_POINT('Ctrl Pts',(7.60520291666221,0.0604213147496031,0.525518178609593));
#7648=CARTESIAN_POINT('Ctrl Pts',(7.58398553332829,0.167119405323871,0.546562317050415));
#7649=CARTESIAN_POINT('Ctrl Pts',(7.49271161354778,0.304100141680242,0.578374094337356));
#7650=CARTESIAN_POINT('Ctrl Pts',(7.35489249545306,0.396201765810716,0.610414265003916));
#7651=CARTESIAN_POINT('Ctrl Pts',(7.1910298751132,0.428986978304214,0.642713211662006));
#7652=CARTESIAN_POINT('Ctrl Pts',(7.02575974448701,0.396160852316168,0.675278092187565));
#7653=CARTESIAN_POINT('Ctrl Pts',(6.88431346091905,0.301887668071453,0.708126241652113));
#7654=CARTESIAN_POINT('Ctrl Pts',(6.78902288535122,0.159380649672213,0.741265999150335));
#7655=CARTESIAN_POINT('Ctrl Pts',(6.75495416610951,-0.0103780765937392,
0.774709380896621));
#7656=CARTESIAN_POINT('Ctrl Pts',(6.78918192236938,-0.181461258490112,0.808462327478204));
#7657=CARTESIAN_POINT('Ctrl Pts',(6.91885908336219,-0.377673922655746,0.853889424408574));
#7658=CARTESIAN_POINT('Ctrl Pts',(7.20977093093628,-0.499893892945984,0.911473809881342));
#7659=CARTESIAN_POINT('Ctrl Pts',(7.5072630858031,-0.377588681747576,0.97014125931953));
#7660=CARTESIAN_POINT('Ctrl Pts',(7.64330562270039,-0.172136868667308,1.01771468839021));
#7661=CARTESIAN_POINT('Ctrl Pts',(7.68999690574486,0.0575070029618808,1.06304113378557));
#7662=CARTESIAN_POINT('Ctrl Pts',(7.58912753114069,0.338304476334369,1.11835008292628));
#7663=CARTESIAN_POINT('Ctrl Pts',(7.28221724491026,0.515932878067702,1.18402351038321));
#7664=CARTESIAN_POINT('Ctrl Pts',(6.95856764177261,0.459622888930078,1.24500482688593));
#7665=CARTESIAN_POINT('Ctrl Pts',(6.75052714561547,0.251003536205887,1.30100630575919));
#7666=CARTESIAN_POINT('Ctrl Pts',(6.6812077153829,-0.00624875161643612,
1.35179871810002));
#7667=CARTESIAN_POINT('Ctrl Pts',(6.75038532199632,-0.2659051370397,1.40293663797005));
#7668=CARTESIAN_POINT('Ctrl Pts',(6.94135907381703,-0.45699229110439,1.45437635262256));
#7669=CARTESIAN_POINT('Ctrl Pts',(7.20350925771528,-0.527428674290956,1.50606241671445));
#7670=CARTESIAN_POINT('Ctrl Pts',(7.466748090342,-0.457001184800688,1.55794289327379));
#7671=CARTESIAN_POINT('Ctrl Pts',(7.65998094988944,-0.263878681039078,1.60996115190039));
#7672=CARTESIAN_POINT('Ctrl Pts',(7.73083750011286,0.000414812515617203,
1.66206037062288));
#7673=CARTESIAN_POINT('Ctrl Pts',(7.65998418428948,0.264828698515665,1.71418231635528));
#7674=CARTESIAN_POINT('Ctrl Pts',(7.46651390251919,0.458227587104288,1.76626886292904));
#7675=CARTESIAN_POINT('Ctrl Pts',(7.20273817979303,0.528826545134251,1.81826192542772));
#7676=CARTESIAN_POINT('Ctrl Pts',(6.93974476704769,0.45822214956276,1.87010491698065));
#7677=CARTESIAN_POINT('Ctrl Pts',(6.74813710185399,0.266377938570576,1.921741689797));
#7678=CARTESIAN_POINT('Ctrl Pts',(6.67836440043136,0.00561142794322326,
1.97312065809906));
#7679=CARTESIAN_POINT('Ctrl Pts',(6.73659880078668,-0.21008625780946,2.0156763602552));
#7680=CARTESIAN_POINT('Ctrl Pts',(6.84232372411288,-0.347442050898008,2.04954129133265));
#7681=CARTESIAN_POINT('Ctrl Pts',(6.9792275847297,-0.452713561295967,2.08327997196431));
#7682=CARTESIAN_POINT('Ctrl Pts',(7.19191177543547,-0.509527438177311,2.1252061938903));
#7683=CARTESIAN_POINT('Ctrl Pts',(7.44484173411992,-0.441538379734714,2.17507245803297));
#7684=CARTESIAN_POINT('Ctrl Pts',(7.62804734440532,-0.257793658448475,2.22446652563413));
#7685=CARTESIAN_POINT('Ctrl Pts',(7.68852622475162,-0.0303820434129393,
2.26927979174901));
#7686=CARTESIAN_POINT('Ctrl Pts',(7.64746376729105,0.174304350641336,2.30962934644072));
#7687=CARTESIAN_POINT('Ctrl Pts',(7.54392328379021,0.329181864553991,2.34563680278534));
#7688=CARTESIAN_POINT('Ctrl Pts',(7.39024341483315,0.431534873640089,2.38133009829314));
#7689=CARTESIAN_POINT('Ctrl Pts',(7.19076283221806,0.47124287783579,2.42063411117922));
#7690=CARTESIAN_POINT('Ctrl Pts',(6.97384163836222,0.412739485800526,2.46340945678261));
#7691=CARTESIAN_POINT('Ctrl Pts',(6.80305475944309,0.241271971337352,2.50949672429145));
#7692=CARTESIAN_POINT('Ctrl Pts',(6.74666636593271,0.0294294813802179,2.55121891282729));
#7693=CARTESIAN_POINT('Ctrl Pts',(6.78501449029175,-0.160618901754849,2.58873736232549));
#7694=CARTESIAN_POINT('Ctrl Pts',(6.91280587361007,-0.353262603670726,2.63334571969464));
#7695=CARTESIAN_POINT('Ctrl Pts',(7.19121233364888,-0.467932358310067,2.68834801025112));
#7696=CARTESIAN_POINT('Ctrl Pts',(7.51997563893116,-0.330454307712312,2.75322227387632));
#7697=CARTESIAN_POINT('Ctrl Pts',(7.63018823078828,-0.0608557124429638,
2.80643316177814));
#7698=CARTESIAN_POINT('Ctrl Pts',(7.58668367923284,0.15294955180044,2.84856125844144));
#7699=CARTESIAN_POINT('Ctrl Pts',(7.4966962551456,0.287961175664924,2.87995407749862));
#7700=CARTESIAN_POINT('Ctrl Pts',(7.36223523212543,0.377561342649274,2.91116449944352));
#7701=CARTESIAN_POINT('Ctrl Pts',(7.20471964510295,0.408886599560007,2.94221245706929));
#7702=CARTESIAN_POINT('Ctrl Pts',(7.04788050645387,0.377567269761301,2.97312030304224));
#7703=CARTESIAN_POINT('Ctrl Pts',(6.91541158632493,0.289068616916533,3.00391053762164));
#7704=CARTESIAN_POINT('Ctrl Pts',(6.82728400624535,0.156959448238268,3.03460541662168));
#7705=CARTESIAN_POINT('Ctrl Pts',(6.79284518780191,-0.0157081775009035,
3.06863471118277));
#7706=CARTESIAN_POINT('Ctrl Pts',(6.8434401979818,-0.205290308031978,3.10599536242566));
#7707=CARTESIAN_POINT('Ctrl Pts',(6.99490561515456,-0.356498560372845,3.14673092879048));
#7708=CARTESIAN_POINT('Ctrl Pts',(7.18440894248466,-0.407388834126994,3.18410164809681));
#7709=CARTESIAN_POINT('Ctrl Pts',(7.35718141101045,-0.372875605837951,3.2181429370676));
#7710=CARTESIAN_POINT('Ctrl Pts',(7.48936817162067,-0.284722401562679,3.24885612739662));
#7711=CARTESIAN_POINT('Ctrl Pts',(7.5779106915596,-0.152141452093539,3.27966780812697));
#7712=CARTESIAN_POINT('Ctrl Pts',(7.61281861301683,0.0222543255280253,3.31404069327135));
#7713=CARTESIAN_POINT('Ctrl Pts',(7.56141031644951,0.215151691836449,3.35205199924827));
#7714=CARTESIAN_POINT('Ctrl Pts',(7.40637132389603,0.370556257164557,3.39382812795649));
#7715=CARTESIAN_POINT('Ctrl Pts',(7.19266579688415,0.427969447901563,3.4359633441571));
#7716=CARTESIAN_POINT('Ctrl Pts',(6.97677320753052,0.370444592935496,3.47849574770186));
#7717=CARTESIAN_POINT('Ctrl Pts',(6.81697021686135,0.211073111139358,3.52146834643601));
#7718=CARTESIAN_POINT('Ctrl Pts',(6.7575107065363,-0.00928891171517924,
3.5649148319991));
#7719=CARTESIAN_POINT('Ctrl Pts',(6.8170432422483,-0.232336689376801,3.60886950546352));
#7720=CARTESIAN_POINT('Ctrl Pts',(6.98197068383346,-0.397821990347889,3.65335335844989));
#7721=CARTESIAN_POINT('Ctrl Pts',(7.21036126557627,-0.459413532859389,3.69838806473246));
#7722=CARTESIAN_POINT('Ctrl Pts',(7.44177728328924,-0.397805970847302,3.74398782560502));
#7723=CARTESIAN_POINT('Ctrl Pts',(7.61359761322389,-0.226593064877533,3.79016109241095));
#7724=CARTESIAN_POINT('Ctrl Pts',(7.67207491746036,-0.00928725692599748,
3.83301473789734));
#7725=CARTESIAN_POINT('Ctrl Pts',(7.63236648003885,0.190570754610721,3.87239027223786));
#7726=CARTESIAN_POINT('Ctrl Pts',(7.5297792392475,0.344489241168015,3.90814703559696));
#7727=CARTESIAN_POINT('Ctrl Pts',(7.37465784873898,0.448244015598285,3.94421635698774));
#7728=CARTESIAN_POINT('Ctrl Pts',(7.19013262440696,0.485169459790194,3.98059224783782));
#7729=CARTESIAN_POINT('Ctrl Pts',(7.00401824150362,0.448227922909911,4.01726483809911));
#7730=CARTESIAN_POINT('Ctrl Pts',(6.84494424822825,0.342162883311033,4.05422370431298));
#7731=CARTESIAN_POINT('Ctrl Pts',(6.7377790395693,0.182076193922272,4.09145704575414));
#7732=CARTESIAN_POINT('Ctrl Pts',(6.6998046109465,-0.00815538506850403,
4.12895008010636));
#7733=CARTESIAN_POINT('Ctrl Pts',(6.73784707742154,-0.199653661771381,4.16668775837162));
#7734=CARTESIAN_POINT('Ctrl Pts',(6.84681665964502,-0.363079625185603,4.20465459753528));
#7735=CARTESIAN_POINT('Ctrl Pts',(7.01102146739613,-0.472832785429877,4.24283021774106));
#7736=CARTESIAN_POINT('Ctrl Pts',(7.20565915814223,-0.511732666532225,4.28119783050688));
#7737=CARTESIAN_POINT('Ctrl Pts',(7.40119766392887,-0.472845697797204,4.31973380172215));
#7738=CARTESIAN_POINT('Ctrl Pts',(7.56768126051989,-0.361809343925003,4.358421783452));
#7739=CARTESIAN_POINT('Ctrl Pts',(7.67922282226515,-0.194826290524122,4.39723061348869));
#7740=CARTESIAN_POINT('Ctrl Pts',(7.70548232719575,-0.0632832490931723,
4.42318248066122));
#7741=CARTESIAN_POINT('Ctrl Pts',(7.70549122320354,0.00271383254598746,
4.43614834370058));
#7742=CARTESIAN_POINT('Ctrl Pts',(7.59425772000626,-0.00245828571258322,
0.562474587627441));
#7743=CARTESIAN_POINT('Ctrl Pts',(7.59425070209586,0.049605111382711,0.572703022803963));
#7744=CARTESIAN_POINT('Ctrl Pts',(7.57357837342717,0.153104623621763,0.593123233412961));
#7745=CARTESIAN_POINT('Ctrl Pts',(7.48570217383275,0.284704689582475,0.623707472840817));
#7746=CARTESIAN_POINT('Ctrl Pts',(7.35420545842841,0.372445934216777,0.654268165611503));
#7747=CARTESIAN_POINT('Ctrl Pts',(7.1991395427834,0.403344341615466,0.684830453955887));
#7748=CARTESIAN_POINT('Ctrl Pts',(7.04394708949579,0.372419394010662,0.715418389788155));
#7749=CARTESIAN_POINT('Ctrl Pts',(6.91208817981755,0.284411118321267,0.746056309925617));
#7750=CARTESIAN_POINT('Ctrl Pts',(6.82386012854329,0.15231772958913,0.776768674224976));
#7751=CARTESIAN_POINT('Ctrl Pts',(6.79256685119417,-0.00407665477365361,
0.80757840707805));
#7752=CARTESIAN_POINT('Ctrl Pts',(6.82398499489209,-0.160818309011226,0.838509649661102));
#7753=CARTESIAN_POINT('Ctrl Pts',(6.94235528076999,-0.339716384151892,0.879941146353341));
#7754=CARTESIAN_POINT('Ctrl Pts',(7.20619100564161,-0.450165980568156,0.932146935825043));
#7755=CARTESIAN_POINT('Ctrl Pts',(7.47426273580571,-0.339694216057503,0.985035363478316));
#7756=CARTESIAN_POINT('Ctrl Pts',(7.5966101933134,-0.154911117746058,1.02782858034605));
#7757=CARTESIAN_POINT('Ctrl Pts',(7.63856043476736,0.0514863727408663,1.0685660742741));
#7758=CARTESIAN_POINT('Ctrl Pts',(7.54796314564829,0.303787110641837,1.11826486854298));
#7759=CARTESIAN_POINT('Ctrl Pts',(7.27183799251809,0.463786696523768,1.17737021220891));
#7760=CARTESIAN_POINT('Ctrl Pts',(6.979509411796,0.413145867177907,1.23244288488132));
#7761=CARTESIAN_POINT('Ctrl Pts',(6.79065030465397,0.224010864274787,1.28324401250854));
#7762=CARTESIAN_POINT('Ctrl Pts',(6.72731021175071,-0.0104347042766862,
1.32953860130455));
#7763=CARTESIAN_POINT('Ctrl Pts',(6.79052629084231,-0.248473274721412,1.37640896854699));
#7764=CARTESIAN_POINT('Ctrl Pts',(6.96651190821311,-0.42488040938561,1.42384890860145));
#7765=CARTESIAN_POINT('Ctrl Pts',(7.20992736454157,-0.490534586687267,1.47184965533436));
#7766=CARTESIAN_POINT('Ctrl Pts',(7.45633551352294,-0.424884919868912,1.52039437044473));
#7767=CARTESIAN_POINT('Ctrl Pts',(7.63882761171195,-0.242897887840433,1.56946170079144));
#7768=CARTESIAN_POINT('Ctrl Pts',(7.70653270701263,0.00848210144412344,
1.61902445509968));
#7769=CARTESIAN_POINT('Ctrl Pts',(7.63882350593151,0.262379273284063,1.66905062455159));
#7770=CARTESIAN_POINT('Ctrl Pts',(7.45162606494433,0.449969447852711,1.71950325371943));
#7771=CARTESIAN_POINT('Ctrl Pts',(7.19376083718428,0.51933449850295,1.77034129362804));
#7772=CARTESIAN_POINT('Ctrl Pts',(6.93400990844331,0.449957716943267,1.82151919554189));
#7773=CARTESIAN_POINT('Ctrl Pts',(6.74275338990983,0.25894867906358,1.87298910713157));
#7774=CARTESIAN_POINT('Ctrl Pts',(6.6721794753372,-0.00344155851917735,
1.92469753383097));
#7775=CARTESIAN_POINT('Ctrl Pts',(6.7311016302344,-0.22275510874685,1.96794489965324));
#7776=CARTESIAN_POINT('Ctrl Pts',(6.8392913285343,-0.363404964177234,2.00260883790367));
#7777=CARTESIAN_POINT('Ctrl Pts',(6.98005366068073,-0.471713783449351,2.03730635823932));
#7778=CARTESIAN_POINT('Ctrl Pts',(7.20024838595684,-0.530815092622124,2.08071930878504));
#7779=CARTESIAN_POINT('Ctrl Pts',(7.4646816222063,-0.460071157751818,2.13283473795993));
#7780=CARTESIAN_POINT('Ctrl Pts',(7.65805360986435,-0.26656205273116,2.18490159146475));
#7781=CARTESIAN_POINT('Ctrl Pts',(7.72260468764345,-0.0248541589762378,
2.23253658214116));
#7782=CARTESIAN_POINT('Ctrl Pts',(7.67876439289767,0.194303019173836,2.27572981817065));
#7783=CARTESIAN_POINT('Ctrl Pts',(7.56739059632431,0.361091093887821,2.31449058128002));
#7784=CARTESIAN_POINT('Ctrl Pts',(7.40112190177162,0.471942442644023,2.3531164111895));
#7785=CARTESIAN_POINT('Ctrl Pts',(7.18420215947571,0.515230280020884,2.39586020388528));
#7786=CARTESIAN_POINT('Ctrl Pts',(6.94699552901196,0.451438689854431,2.4426223367052));
#7787=CARTESIAN_POINT('Ctrl Pts',(6.75916567417327,0.263096514005349,2.493274778268));
#7788=CARTESIAN_POINT('Ctrl Pts',(6.69679959781039,0.0292602423063323,2.53933073840707));
#7789=CARTESIAN_POINT('Ctrl Pts',(6.73922836906146,-0.181202753664555,2.5808764986312));
#7790=CARTESIAN_POINT('Ctrl Pts',(6.88098489158572,-0.395007257634639,2.6303774480251));
#7791=CARTESIAN_POINT('Ctrl Pts',(7.19061459426917,-0.522666325469509,2.69155654194586));
#7792=CARTESIAN_POINT('Ctrl Pts',(7.55656339289891,-0.369582360088882,2.76376828329337));
#7793=CARTESIAN_POINT('Ctrl Pts',(7.67882740451396,-0.0699592370443201,
2.8228934499334));
#7794=CARTESIAN_POINT('Ctrl Pts',(7.63057360286556,0.166780390817294,2.86954705222393));
#7795=CARTESIAN_POINT('Ctrl Pts',(7.53116289386047,0.315835424321569,2.90421442771358));
#7796=CARTESIAN_POINT('Ctrl Pts',(7.38316944888177,0.414366909131833,2.93855849946981));
#7797=CARTESIAN_POINT('Ctrl Pts',(7.21055140032512,0.448612501483557,2.97258326216516));
#7798=CARTESIAN_POINT('Ctrl Pts',(7.03953063478659,0.414371602633185,3.00629223766092));
#7799=CARTESIAN_POINT('Ctrl Pts',(6.89590035707824,0.318294406438298,3.03969251978853));
#7800=CARTESIAN_POINT('Ctrl Pts',(6.80097093648036,0.175798229922379,3.07279237357639));
#7801=CARTESIAN_POINT('Ctrl Pts',(6.76420446601918,-0.00918969341029978,
3.10924534420836));
#7802=CARTESIAN_POINT('Ctrl Pts',(6.81822428058444,-0.21055882798918,3.14894909070633));
#7803=CARTESIAN_POINT('Ctrl Pts',(6.97773218443497,-0.36935136486928,3.19179489876111));
#7804=CARTESIAN_POINT('Ctrl Pts',(7.17495518145593,-0.422006833075381,3.23067901466676));
#7805=CARTESIAN_POINT('Ctrl Pts',(7.35286337729078,-0.386309768778915,3.26574476462206));
#7806=CARTESIAN_POINT('Ctrl Pts',(7.48774464276126,-0.296188781696453,3.29710501689698));
#7807=CARTESIAN_POINT('Ctrl Pts',(7.57721901263156,-0.161961982729025,3.32828683420642));
#7808=CARTESIAN_POINT('Ctrl Pts',(7.61206314196752,0.0129508069889947,3.36275642269021));
#7809=CARTESIAN_POINT('Ctrl Pts',(7.56075482794487,0.204285379935896,3.40048407841003));
#7810=CARTESIAN_POINT('Ctrl Pts',(7.40850398946938,0.356408978558438,3.44145294697141));
#7811=CARTESIAN_POINT('Ctrl Pts',(7.20135390499387,0.41173394168823,3.48228578202979));
#7812=CARTESIAN_POINT('Ctrl Pts',(6.99457227847817,0.356315965170544,3.52304732856917));
#7813=CARTESIAN_POINT('Ctrl Pts',(6.84328577478245,0.205035111445078,3.56379125585673));
#7814=CARTESIAN_POINT('Ctrl Pts',(6.7877374954679,-0.00186586115036843,
3.60457861601043));
#7815=CARTESIAN_POINT('Ctrl Pts',(6.84333329257615,-0.209237336684351,3.64546113573529));
#7816=CARTESIAN_POINT('Ctrl Pts',(6.99562840241749,-0.361741579815771,3.68650281084151));
#7817=CARTESIAN_POINT('Ctrl Pts',(7.20485782405896,-0.417973379258145,3.72775549001309));
#7818=CARTESIAN_POINT('Ctrl Pts',(7.41548973555594,-0.361739190165172,3.76927272327787));
#7819=CARTESIAN_POINT('Ctrl Pts',(7.5710498247318,-0.206554713249447,3.81110431032449));
#7820=CARTESIAN_POINT('Ctrl Pts',(7.62374712773981,-0.0104230426211467,
3.84978234597979));
#7821=CARTESIAN_POINT('Ctrl Pts',(7.58796837467257,0.169522444365365,3.88523795926289));
#7822=CARTESIAN_POINT('Ctrl Pts',(7.49570620913085,0.307926121393348,3.91739357370391));
#7823=CARTESIAN_POINT('Ctrl Pts',(7.35630624460567,0.401161458520253,3.94980772489261));
#7824=CARTESIAN_POINT('Ctrl Pts',(7.19048793327558,0.434350296220375,3.98249611828477));
#7825=CARTESIAN_POINT('Ctrl Pts',(7.02313732463905,0.401152548579443,4.01547086689915));
#7826=CARTESIAN_POINT('Ctrl Pts',(6.87991827712017,0.305692036987412,4.04874191834322));
#7827=CARTESIAN_POINT('Ctrl Pts',(6.78324141246895,0.161344852331597,4.08231922585133));
#7828=CARTESIAN_POINT('Ctrl Pts',(6.74886677350852,-0.0105999920447858,
4.11620911872423));
#7829=CARTESIAN_POINT('Ctrl Pts',(6.78329499176258,-0.18420466099095,4.15041748648745));
#7830=CARTESIAN_POINT('Ctrl Pts',(6.88234563382671,-0.332882015591908,4.18494784070123));
#7831=CARTESIAN_POINT('Ctrl Pts',(7.03222479883265,-0.433150934079335,4.21980148929331));
#7832=CARTESIAN_POINT('Ctrl Pts',(7.21066650576015,-0.468899513976003,4.25497951717241));
#7833=CARTESIAN_POINT('Ctrl Pts',(7.39081341647505,-0.433166214217135,4.29047687728664));
#7834=CARTESIAN_POINT('Ctrl Pts',(7.54500124432846,-0.330435384103034,4.32629673150718));
#7835=CARTESIAN_POINT('Ctrl Pts',(7.648911736291,-0.175068311549345,4.36241691197868));
#7836=CARTESIAN_POINT('Ctrl Pts',(7.67356138220208,-0.051891031334385,4.38672007785258));
#7837=CARTESIAN_POINT('Ctrl Pts',(7.67356972993859,0.010038573569273,4.39888683970507));
#7838=CARTESIAN_POINT('Ctrl Pts',(7.6251463906065,-0.00995933879406772,
0.600676626589758));
#7839=CARTESIAN_POINT('Ctrl Pts',(7.62513886057627,0.0459032942528346,0.611651464053095));
#7840=CARTESIAN_POINT('Ctrl Pts',(7.60292290623068,0.156870790432269,0.633544848495396));
#7841=CARTESIAN_POINT('Ctrl Pts',(7.50931870776666,0.296831365590117,0.666081330908944));
#7842=CARTESIAN_POINT('Ctrl Pts',(7.37036934701443,0.389419470623286,0.698359968830145));
#7843=CARTESIAN_POINT('Ctrl Pts',(7.20784862587356,0.421674331381802,0.730381922456915));
#7844=CARTESIAN_POINT('Ctrl Pts',(7.04659254578026,0.389405737732574,0.762169124409136));
#7845=CARTESIAN_POINT('Ctrl Pts',(6.91079445014922,0.298603087234844,0.793736135243985));
#7846=CARTESIAN_POINT('Ctrl Pts',(6.8207979343427,0.163604010555256,0.825103242993061));
#7847=CARTESIAN_POINT('Ctrl Pts',(6.78926618396683,0.00524540576184069,
0.856289595657219));
#7848=CARTESIAN_POINT('Ctrl Pts',(6.82091005115504,-0.151956334869631,0.887316325014752));
#7849=CARTESIAN_POINT('Ctrl Pts',(6.93880442644738,-0.329744857889583,0.928502477696562));
#7850=CARTESIAN_POINT('Ctrl Pts',(7.19794632806152,-0.437170841618844,0.97969295172908));
#7851=CARTESIAN_POINT('Ctrl Pts',(7.45594932305352,-0.329838555678054,1.03065941290864));
#7852=CARTESIAN_POINT('Ctrl Pts',(7.57223630638577,-0.15388196293264,1.07139312359183));
#7853=CARTESIAN_POINT('Ctrl Pts',(7.61173195193373,0.0411613828711062,1.10987247621873));
#7854=CARTESIAN_POINT('Ctrl Pts',(7.52649198341673,0.276889962424743,1.15632864381613));
#7855=CARTESIAN_POINT('Ctrl Pts',(7.27100861906712,0.424277981015224,1.21095498218268));
#7856=CARTESIAN_POINT('Ctrl Pts',(7.00347558016671,0.377525264901119,1.26136760852975));
#7857=CARTESIAN_POINT('Ctrl Pts',(6.83192597243994,0.205463838889712,1.30754770952591));
#7858=CARTESIAN_POINT('Ctrl Pts',(6.77471877393629,-0.00671405179287721,
1.34943621263325));
#7859=CARTESIAN_POINT('Ctrl Pts',(6.83181225604176,-0.221332534887357,1.39169859189476));
#7860=CARTESIAN_POINT('Ctrl Pts',(6.99015954735038,-0.379977992431842,1.43437163868664));
#7861=CARTESIAN_POINT('Ctrl Pts',(7.20886960086134,-0.438945066985825,1.47749887936028));
#7862=CARTESIAN_POINT('Ctrl Pts',(7.43024747996125,-0.379973659956208,1.52111182668763));
#7863=CARTESIAN_POINT('Ctrl Pts',(7.59439894652586,-0.216337713478778,1.56524030048575));
#7864=CARTESIAN_POINT('Ctrl Pts',(7.65548722497565,0.0101858356141963,1.60990738944098));
#7865=CARTESIAN_POINT('Ctrl Pts',(7.59438357985085,0.239727786394584,1.65513131383826));
#7866=CARTESIAN_POINT('Ctrl Pts',(7.42458127262742,0.410079670414055,1.70092433297305));
#7867=CARTESIAN_POINT('Ctrl Pts',(7.1894457064806,0.473501570956881,1.74729294719369));
#7868=CARTESIAN_POINT('Ctrl Pts',(6.95114935036374,0.410054983182796,1.79423785660882));
#7869=CARTESIAN_POINT('Ctrl Pts',(6.77444906673486,0.233888130858127,1.8417535579876));
#7870=CARTESIAN_POINT('Ctrl Pts',(6.70860511145662,-0.00997119589789413,
1.8898294385356));
#7871=CARTESIAN_POINT('Ctrl Pts',(6.76359263836854,-0.215478331596112,1.93034449371185));
#7872=CARTESIAN_POINT('Ctrl Pts',(6.86552920528386,-0.348073042081005,1.96301641877778));
#7873=CARTESIAN_POINT('Ctrl Pts',(6.99871512481987,-0.450608012381444,1.99585725873467));
#7874=CARTESIAN_POINT('Ctrl Pts',(7.20840141309144,-0.50713987259909,2.03721833824704));
#7875=CARTESIAN_POINT('Ctrl Pts',(7.46261403294825,-0.439449176754183,2.08730887227053));
#7876=CARTESIAN_POINT('Ctrl Pts',(7.65043036508478,-0.251969993404681,2.13782457411003));
#7877=CARTESIAN_POINT('Ctrl Pts',(7.71393504862941,-0.0153445846184741,
2.1844803492873));
#7878=CARTESIAN_POINT('Ctrl Pts',(7.67080165909933,0.201106000343718,2.22713471421714));
#7879=CARTESIAN_POINT('Ctrl Pts',(7.56014087497921,0.367078706762164,2.2656927101989));
#7880=CARTESIAN_POINT('Ctrl Pts',(7.39362722575602,0.47826661439383,2.30439640224526));
#7881=CARTESIAN_POINT('Ctrl Pts',(7.17474883695495,0.5221088112285,2.34753793394624));
#7882=CARTESIAN_POINT('Ctrl Pts',(6.93323485822253,0.457485550857918,2.39514037933818));
#7883=CARTESIAN_POINT('Ctrl Pts',(6.73999704643146,0.264200773821966,2.44718908940685));
#7884=CARTESIAN_POINT('Ctrl Pts',(6.6750106891604,0.0217479615274458,2.49496582442984));
#7885=CARTESIAN_POINT('Ctrl Pts',(6.71923769435572,-0.198307386666359,2.53840100430929));
#7886=CARTESIAN_POINT('Ctrl Pts',(6.86820572152663,-0.423361666552716,2.59049654373951));
#7887=CARTESIAN_POINT('Ctrl Pts',(7.19683451438197,-0.559762287000885,2.65550316184341));
#7888=CARTESIAN_POINT('Ctrl Pts',(7.59061985625878,-0.39609337580252,2.73313735372284));
#7889=CARTESIAN_POINT('Ctrl Pts',(7.72404765466645,-0.0708376341742968,
2.79737041159043));
#7890=CARTESIAN_POINT('Ctrl Pts',(7.67138895603303,0.188103473826818,2.84838979927756));
#7891=CARTESIAN_POINT('Ctrl Pts',(7.56230591732181,0.35178346601004,2.88645331216893));
#7892=CARTESIAN_POINT('Ctrl Pts',(7.39927679222285,0.46041116731156,2.92429660886102));
#7893=CARTESIAN_POINT('Ctrl Pts',(7.2085057862945,0.498313460595825,2.96190202559112));
#7894=CARTESIAN_POINT('Ctrl Pts',(7.01899650553946,0.460419063486977,2.99925417953252));
#7895=CARTESIAN_POINT('Ctrl Pts',(6.8595074148951,0.353776728734024,3.03633740791343));
#7896=CARTESIAN_POINT('Ctrl Pts',(6.75393754656612,0.195352351115091,3.07314022143174));
#7897=CARTESIAN_POINT('Ctrl Pts',(6.71300839906166,-0.0105024876967131,
3.11370534962017));
#7898=CARTESIAN_POINT('Ctrl Pts',(6.77313540889629,-0.23465187277845,3.1578981321776));
#7899=CARTESIAN_POINT('Ctrl Pts',(6.9505773913537,-0.411233490999672,3.2055512312233));
#7900=CARTESIAN_POINT('Ctrl Pts',(7.16952277235119,-0.469618095917656,3.24871160420247));
#7901=CARTESIAN_POINT('Ctrl Pts',(7.36645966236824,-0.430046136418131,3.28752910700568));
#7902=CARTESIAN_POINT('Ctrl Pts',(7.51530337347556,-0.330531283613474,3.322140113292));
#7903=CARTESIAN_POINT('Ctrl Pts',(7.6136393067511,-0.182885406541807,3.35642864300427));
#7904=CARTESIAN_POINT('Ctrl Pts',(7.6517119731009,0.00866863156965702,3.39417116601774));
#7905=CARTESIAN_POINT('Ctrl Pts',(7.59566292791954,0.216926348779987,3.43523841335543));
#7906=CARTESIAN_POINT('Ctrl Pts',(7.43098841093127,0.381112304766534,3.47949475317577));
#7907=CARTESIAN_POINT('Ctrl Pts',(7.20902257822881,0.440109346407386,3.52323182285004));
#7908=CARTESIAN_POINT('Ctrl Pts',(6.98969677272196,0.381025501634275,3.56647300951898));
#7909=CARTESIAN_POINT('Ctrl Pts',(6.83104480220145,0.221934930884199,3.60925399866409));
#7910=CARTESIAN_POINT('Ctrl Pts',(6.77366702945068,0.00694265778365469,
3.6516094283646));
#7911=CARTESIAN_POINT('Ctrl Pts',(6.8310824464219,-0.205902622087142,3.6935863577146));
#7912=CARTESIAN_POINT('Ctrl Pts',(6.98586160732495,-0.360410071323003,3.73522365094446));
#7913=CARTESIAN_POINT('Ctrl Pts',(7.19571361575979,-0.416451275528931,3.77657387332006));
#7914=CARTESIAN_POINT('Ctrl Pts',(7.40425474387956,-0.360423855799516,3.81768805486677));
#7915=CARTESIAN_POINT('Ctrl Pts',(7.5562630491962,-0.208304194865644,3.85862159368099));
#7916=CARTESIAN_POINT('Ctrl Pts',(7.60695606004407,-0.0185100802651633,
3.89602785586108));
#7917=CARTESIAN_POINT('Ctrl Pts',(7.57254113144743,0.153827290746397,3.92998748438201));
#7918=CARTESIAN_POINT('Ctrl Pts',(7.48477263414739,0.28527139080477,3.96053536270553));
#7919=CARTESIAN_POINT('Ctrl Pts',(7.35326159780128,0.373088001773748,3.99109827766809));
#7920=CARTESIAN_POINT('Ctrl Pts',(7.19801139434241,0.404051485210006,4.02169520823128));
#7921=CARTESIAN_POINT('Ctrl Pts',(7.04242854792053,0.373082428795767,4.05235230289711));
#7922=CARTESIAN_POINT('Ctrl Pts',(6.91013509296653,0.284793306662795,4.08309464265432));
#7923=CARTESIAN_POINT('Ctrl Pts',(6.82137789485868,0.152112705303776,4.11394287723527));
#7924=CARTESIAN_POINT('Ctrl Pts',(6.79002667088262,-0.00509640153436752,
4.14492325438676));
#7925=CARTESIAN_POINT('Ctrl Pts',(6.82142807903689,-0.163089310650938,4.17605557225883));
#7926=CARTESIAN_POINT('Ctrl Pts',(6.9112855133859,-0.297866472185936,4.20736152086343));
#7927=CARTESIAN_POINT('Ctrl Pts',(7.04678082670187,-0.388454515500582,4.23886139687883));
#7928=CARTESIAN_POINT('Ctrl Pts',(7.20767263671213,-0.420652573613419,4.27057542931576));
#7929=CARTESIAN_POINT('Ctrl Pts',(7.36979084225692,-0.388467264966068,4.30251884135981));
#7930=CARTESIAN_POINT('Ctrl Pts',(7.50837984637881,-0.296115525357199,4.3347137808459));
#7931=CARTESIAN_POINT('Ctrl Pts',(7.60172624083291,-0.156526571753314,4.36716218083725));
#7932=CARTESIAN_POINT('Ctrl Pts',(7.62387694790615,-0.0458686559730776,
4.38899381459629));
#7933=CARTESIAN_POINT('Ctrl Pts',(7.62388445692499,0.00983872883570376,
4.39993815188776));
#7934=CARTESIAN_POINT('Ctrl Pts',(7.67479866661154,-0.00992467619824002,
0.600534259038771));
#7935=CARTESIAN_POINT('Ctrl Pts',(7.67479029797541,0.0521592777126054,0.612731344390634));
#7936=CARTESIAN_POINT('Ctrl Pts',(7.6500767264732,0.175648933321932,0.637096797205508));
#7937=CARTESIAN_POINT('Ctrl Pts',(7.54588794825347,0.331423934572361,0.673313288688549));
#7938=CARTESIAN_POINT('Ctrl Pts',(7.39127793836307,0.434435241125366,0.709231481896876));
#7939=CARTESIAN_POINT('Ctrl Pts',(7.21062039986564,0.470261715425624,0.744828861653363));
#7940=CARTESIAN_POINT('Ctrl Pts',(7.03167221168909,0.434417722011693,0.780107884329232));
#7941=CARTESIAN_POINT('Ctrl Pts',(6.88134081087794,0.333835280809163,0.815063046988659));
#7942=CARTESIAN_POINT('Ctrl Pts',(6.78203321069345,0.184769764667609,0.849694716646961));
#7943=CARTESIAN_POINT('Ctrl Pts',(6.74742301017565,0.0105515865458462,0.884003789334016));
#7944=CARTESIAN_POINT('Ctrl Pts',(6.7821506919055,-0.161614361391387,0.917993137651611));
#7945=CARTESIAN_POINT('Ctrl Pts',(6.91079450905087,-0.35538315192201,0.962892520561796));
#7946=CARTESIAN_POINT('Ctrl Pts',(7.19125186153526,-0.470870066280229,1.01824785147389));
#7947=CARTESIAN_POINT('Ctrl Pts',(7.46622186533978,-0.355583864325095,1.07263464146893));
#7948=CARTESIAN_POINT('Ctrl Pts',(7.58869616833744,-0.169899793625554,1.11561531576428));
#7949=CARTESIAN_POINT('Ctrl Pts',(7.62989084686889,0.0343026557437226,1.1558927821855));
#7950=CARTESIAN_POINT('Ctrl Pts',(7.54102211851986,0.278002087645062,1.20397798366483));
#7951=CARTESIAN_POINT('Ctrl Pts',(7.28038899375006,0.427368120216494,1.25963095207772));
#7952=CARTESIAN_POINT('Ctrl Pts',(7.01236273858795,0.379779461323442,1.31016266895165));
#7953=CARTESIAN_POINT('Ctrl Pts',(6.84312930177798,0.209454684258967,1.35581730583755));
#7954=CARTESIAN_POINT('Ctrl Pts',(6.7875566642785,0.00215073089889336,1.39673552660572));
#7955=CARTESIAN_POINT('Ctrl Pts',(6.84299249099257,-0.204955992335496,1.43753752961745));
#7956=CARTESIAN_POINT('Ctrl Pts',(6.99438077830621,-0.356203083369992,1.47828922226758));
#7957=CARTESIAN_POINT('Ctrl Pts',(7.20108707217728,-0.411642052898573,1.51904138345725));
#7958=CARTESIAN_POINT('Ctrl Pts',(7.40815060417183,-0.356215475951744,1.55985546395848));
#7959=CARTESIAN_POINT('Ctrl Pts',(7.56022255433633,-0.204292849888386,1.6007875102571));
#7960=CARTESIAN_POINT('Ctrl Pts',(7.6162350845383,0.00419615192836477,1.64189449134062));
#7961=CARTESIAN_POINT('Ctrl Pts',(7.56022316647258,0.213929952633467,1.68323060525625));
#7962=CARTESIAN_POINT('Ctrl Pts',(7.40582151724235,0.368627873830385,1.72484818318265));
#7963=CARTESIAN_POINT('Ctrl Pts',(7.19309620708298,0.42588980315725,1.7667963623234));
#7964=CARTESIAN_POINT('Ctrl Pts',(6.97829166980193,0.368617545064421,1.80912125797898));
#7965=CARTESIAN_POINT('Ctrl Pts',(6.81938158401184,0.210124736402539,1.85186448361653));
#7966=CARTESIAN_POINT('Ctrl Pts',(6.76022871604125,-0.00899134529255971,
1.89506476553187));
#7967=CARTESIAN_POINT('Ctrl Pts',(6.80961939806014,-0.193661886224269,1.93147173029523));
#7968=CARTESIAN_POINT('Ctrl Pts',(6.90128880494812,-0.312919191995625,1.96085533209598));
#7969=CARTESIAN_POINT('Ctrl Pts',(7.02116296768677,-0.405217714775714,1.99041541019261));
#7970=CARTESIAN_POINT('Ctrl Pts',(7.2101902287687,-0.456256683551471,2.0277044964254));
#7971=CARTESIAN_POINT('Ctrl Pts',(7.44013817723507,-0.39514737391709,2.07300715398026));
#7972=CARTESIAN_POINT('Ctrl Pts',(7.61080888298339,-0.224999902344798,2.11888000691673));
#7973=CARTESIAN_POINT('Ctrl Pts',(7.66892725315019,-0.00908328955551635,
2.16145591840512));
#7974=CARTESIAN_POINT('Ctrl Pts',(7.62945122739719,0.189485836845824,2.20058130338214));
#7975=CARTESIAN_POINT('Ctrl Pts',(7.5275438271907,0.342497311992806,2.23611409854177));
#7976=CARTESIAN_POINT('Ctrl Pts',(7.37334783976495,0.445576027600189,2.27196416979245));
#7977=CARTESIAN_POINT('Ctrl Pts',(7.16952106168795,0.486525787486152,2.31214252862709));
#7978=CARTESIAN_POINT('Ctrl Pts',(6.94300344132289,0.42617239887457,2.35676948181569));
#7979=CARTESIAN_POINT('Ctrl Pts',(6.76011882687655,0.243647090636264,2.40597173678973));
#7980=CARTESIAN_POINT('Ctrl Pts',(6.69787591763812,0.0125389329026939,2.45151668259076));
#7981=CARTESIAN_POINT('Ctrl Pts',(6.74025578358462,-0.198992447969517,2.49325466511179));
#7982=CARTESIAN_POINT('Ctrl Pts',(6.88420849211811,-0.41683400693851,2.54365885019681));
#7983=CARTESIAN_POINT('Ctrl Pts',(7.20519838849559,-0.551093588719466,2.60722003202361));
#7984=CARTESIAN_POINT('Ctrl Pts',(7.59637091882833,-0.389875109666415,2.68423239344864));
#7985=CARTESIAN_POINT('Ctrl Pts',(7.73161202088386,-0.0627950541721369,
2.74887995748231));
#7986=CARTESIAN_POINT('Ctrl Pts',(7.67821621404377,0.200815500874292,2.800795072092));
#7987=CARTESIAN_POINT('Ctrl Pts',(7.56652799154434,0.368635913177726,2.8398029009376));
#7988=CARTESIAN_POINT('Ctrl Pts',(7.39832631725958,0.480881956369855,2.87885956424108));
#7989=CARTESIAN_POINT('Ctrl Pts',(7.20007842418665,0.520408671552025,2.91794004656954));
#7990=CARTESIAN_POINT('Ctrl Pts',(7.00175111169393,0.48088156284492,2.95701986564842));
#7991=CARTESIAN_POINT('Ctrl Pts',(6.83369430575371,0.368667574968921,2.99607525105644));
#7992=CARTESIAN_POINT('Ctrl Pts',(6.72169316671637,0.200802407429077,3.03507982827121));
#7993=CARTESIAN_POINT('Ctrl Pts',(6.6779145850631,-0.0187059625261386,3.0783398943622));
#7994=CARTESIAN_POINT('Ctrl Pts',(6.74223823189394,-0.259425539513033,3.12578113707604));
#7995=CARTESIAN_POINT('Ctrl Pts',(6.93397723224707,-0.450570898703853,3.17731127091177));
#7996=CARTESIAN_POINT('Ctrl Pts',(7.1722647119663,-0.51431424077328,3.22429041505122));
#7997=CARTESIAN_POINT('Ctrl Pts',(7.38777183560922,-0.471096886879066,3.26675960479394));
#7998=CARTESIAN_POINT('Ctrl Pts',(7.55131219363285,-0.361840084601825,3.30477820464692));
#7999=CARTESIAN_POINT('Ctrl Pts',(7.65975942831194,-0.199115335498351,3.34257273329541));
#8000=CARTESIAN_POINT('Ctrl Pts',(7.70191108793092,0.0126587082651895,3.38430173234848));
#8001=CARTESIAN_POINT('Ctrl Pts',(7.63984171392963,0.24359688777398,3.42983440925146));
#8002=CARTESIAN_POINT('Ctrl Pts',(7.45686243056377,0.426111652973154,3.47901961565964));
#8003=CARTESIAN_POINT('Ctrl Pts',(7.20986017068608,0.491783017499628,3.52768953921784));
#8004=CARTESIAN_POINT('Ctrl Pts',(6.96574932197927,0.42600252056967,3.57581950032201));
#8005=CARTESIAN_POINT('Ctrl Pts',(6.78936748485555,0.249056980614626,3.62339237126234));
#8006=CARTESIAN_POINT('Ctrl Pts',(6.72578712981547,0.0104579783117708,3.6703970656946));
#8007=CARTESIAN_POINT('Ctrl Pts',(6.78941191873306,-0.22492423847484,3.71682678335395));
#8008=CARTESIAN_POINT('Ctrl Pts',(6.9599707009394,-0.394951542887189,3.76268295455715));
#8009=CARTESIAN_POINT('Ctrl Pts',(7.18982623952553,-0.456130340124368,3.80797027228821));
#8010=CARTESIAN_POINT('Ctrl Pts',(7.41661698388298,-0.394964306963868,3.8527010569297));
#8011=CARTESIAN_POINT('Ctrl Pts',(7.58051422722045,-0.230580202674474,3.89689197253134));
#8012=CARTESIAN_POINT('Ctrl Pts',(7.63450803247875,-0.0274292607074651,
3.9369279396462));
#8013=CARTESIAN_POINT('Ctrl Pts',(7.59785383835248,0.155398772912859,3.97296600933491));
#8014=CARTESIAN_POINT('Ctrl Pts',(7.50532059797367,0.293739897374131,4.00514140052698));
#8015=CARTESIAN_POINT('Ctrl Pts',(7.36788217274004,0.385354559507254,4.03706791208184));
#8016=CARTESIAN_POINT('Ctrl Pts',(7.2070357335576,0.417288319469129,4.06876724211276));
#8017=CARTESIAN_POINT('Ctrl Pts',(7.04729419715336,0.385346151743235,4.10025531214439));
#8018=CARTESIAN_POINT('Ctrl Pts',(6.9127169339232,0.295357215095775,4.13155072863576));
#8019=CARTESIAN_POINT('Ctrl Pts',(6.8233007999502,0.16142663300187,4.16267626015357));
#8020=CARTESIAN_POINT('Ctrl Pts',(6.79210610834504,0.00424230951374864,
4.19365003347802));
#8021=CARTESIAN_POINT('Ctrl Pts',(6.82335152241767,-0.152245393365304,4.22449627052708));
#8022=CARTESIAN_POINT('Ctrl Pts',(6.91170118225541,-0.284497538555319,4.2552382224001));
#8023=CARTESIAN_POINT('Ctrl Pts',(7.0436328417148,-0.372545139247727,4.28589810740223));
#8024=CARTESIAN_POINT('Ctrl Pts',(7.19889934274857,-0.403485302426958,4.31650036598566));
#8025=CARTESIAN_POINT('Ctrl Pts',(7.35398823305083,-0.372573048928812,4.34706944683436));
#8026=CARTESIAN_POINT('Ctrl Pts',(7.48547509251604,-0.284834315514199,4.37762904432927));
#8027=CARTESIAN_POINT('Ctrl Pts',(7.57331921955373,-0.153270744978136,4.4082049409292));
#8028=CARTESIAN_POINT('Ctrl Pts',(7.59397776075199,-0.0498297474199503,
4.42861399797485));
#8029=CARTESIAN_POINT('Ctrl Pts',(7.59398477416145,0.00220084515175098,
4.43883598840815));
#8030=CARTESIAN_POINT('Ctrl Pts',(7.70589891767588,-0.00245359116008025,
0.562527291052974));
#8031=CARTESIAN_POINT('Ctrl Pts',(7.70589001475021,0.0635940679486153,0.57550309050989));
#8032=CARTESIAN_POINT('Ctrl Pts',(7.67960751727991,0.195246334704192,0.601476943597424));
#8033=CARTESIAN_POINT('Ctrl Pts',(7.56794704817328,0.362402774430045,0.640326865453731));
#8034=CARTESIAN_POINT('Ctrl Pts',(7.40125695808951,0.473579993253837,0.679063145032516));
#8035=CARTESIAN_POINT('Ctrl Pts',(7.20543306486306,0.512518883001897,0.71765425115707));
#8036=CARTESIAN_POINT('Ctrl Pts',(7.01048476585089,0.47356858176727,0.75608392728287));
#8037=CARTESIAN_POINT('Ctrl Pts',(6.84596393699636,0.363597944823763,0.794327562675024));
#8038=CARTESIAN_POINT('Ctrl Pts',(6.73681549467478,0.199907515410705,0.832368570550477));
#8039=CARTESIAN_POINT('Ctrl Pts',(6.69859516683231,0.00788873917180853,
0.870185654844328));
#8040=CARTESIAN_POINT('Ctrl Pts',(6.73693840908256,-0.182462612245687,0.907764070762306));
#8041=CARTESIAN_POINT('Ctrl Pts',(6.87944326222088,-0.397259890598946,0.957526324120129));
#8042=CARTESIAN_POINT('Ctrl Pts',(7.19112164610969,-0.52580429954268,1.019055817578));
#8043=CARTESIAN_POINT('Ctrl Pts',(7.49727265912014,-0.397485516076704,1.07960188006838));
#8044=CARTESIAN_POINT('Ctrl Pts',(7.63350319008322,-0.190883659121824,1.12741548650668));
#8045=CARTESIAN_POINT('Ctrl Pts',(7.67926654816378,0.0360593370384181,1.17217372176293));
#8046=CARTESIAN_POINT('Ctrl Pts',(7.58056509985602,0.306162895092056,1.2254647678339));
#8047=CARTESIAN_POINT('Ctrl Pts',(7.29294272175984,0.470562172818316,1.28683106259674));
#8048=CARTESIAN_POINT('Ctrl Pts',(6.99954581718474,0.418054042402384,1.34215587872395));
#8049=CARTESIAN_POINT('Ctrl Pts',(6.81596154951457,0.232892123969687,1.39172465766909));
#8050=CARTESIAN_POINT('Ctrl Pts',(6.75631856140084,0.00947775492955636,
1.43580133529387));
#8051=CARTESIAN_POINT('Ctrl Pts',(6.8157947547332,-0.211634317055903,1.4793685868871));
#8052=CARTESIAN_POINT('Ctrl Pts',(6.97609023807819,-0.371345558222595,1.52244706084194));
#8053=CARTESIAN_POINT('Ctrl Pts',(7.1924649342669,-0.429050195429467,1.56507891751011));
#8054=CARTESIAN_POINT('Ctrl Pts',(7.4066375984947,-0.37137171946741,1.6072994439806));
#8055=CARTESIAN_POINT('Ctrl Pts',(7.56193269569475,-0.215745610884436,1.64915326420547));
#8056=CARTESIAN_POINT('Ctrl Pts',(7.61820626718149,-0.00494726647780665,
1.69068645168105));
#8057=CARTESIAN_POINT('Ctrl Pts',(7.561944028498,0.204380228806823,1.7319494515681));
#8058=CARTESIAN_POINT('Ctrl Pts',(7.40938473246838,0.356749091593267,1.77299486946184));
#8059=CARTESIAN_POINT('Ctrl Pts',(7.20192341170518,0.41224876158547,1.81387806697088));
#8060=CARTESIAN_POINT('Ctrl Pts',(6.99500876965101,0.35674779749565,1.85465522832279));
#8061=CARTESIAN_POINT('Ctrl Pts',(6.84376585084722,0.205473612051122,1.89538529487664));
#8062=CARTESIAN_POINT('Ctrl Pts',(6.78825237597385,-0.00128361409126172,
1.93612397126094));
#8063=CARTESIAN_POINT('Ctrl Pts',(6.83460167043985,-0.173751988890528,1.97013317734193));
#8064=CARTESIAN_POINT('Ctrl Pts',(6.91971539174711,-0.284417737520675,1.99740528786609));
#8065=CARTESIAN_POINT('Ctrl Pts',(7.030558325938,-0.369712270987243,2.02472860539297));
#8066=CARTESIAN_POINT('Ctrl Pts',(7.20432462750735,-0.416450035553709,2.05899164095769));
#8067=CARTESIAN_POINT('Ctrl Pts',(7.41421871524057,-0.360487797716962,2.10035061982331));
#8068=CARTESIAN_POINT('Ctrl Pts',(7.56905709734982,-0.20590418677377,2.14199286175633));
#8069=CARTESIAN_POINT('Ctrl Pts',(7.62148773641759,-0.0107077758477395,
2.1804754775963));
#8070=CARTESIAN_POINT('Ctrl Pts',(7.58586473971553,0.168272748684638,2.215741820189));
#8071=CARTESIAN_POINT('Ctrl Pts',(7.49414435933883,0.305939339339139,2.2477146319058));
#8072=CARTESIAN_POINT('Ctrl Pts',(7.35554181248979,0.398575104482043,2.27993674611506));
#8073=CARTESIAN_POINT('Ctrl Pts',(7.1724244687894,0.435355812617659,2.31603381922843));
#8074=CARTESIAN_POINT('Ctrl Pts',(6.96887901773368,0.381138200319487,2.35613647030697));
#8075=CARTESIAN_POINT('Ctrl Pts',(6.80429530787655,0.216951871529364,2.40040714688527));
#8076=CARTESIAN_POINT('Ctrl Pts',(6.74808716941278,0.00854379166712036,
2.44148821315331));
#8077=CARTESIAN_POINT('Ctrl Pts',(6.78637616860293,-0.182801008849154,2.47924298930385));
#8078=CARTESIAN_POINT('Ctrl Pts',(6.91689579762816,-0.380440663799344,2.52497536795987));
#8079=CARTESIAN_POINT('Ctrl Pts',(7.20943026727739,-0.503307468048506,2.58295046852016));
#8080=CARTESIAN_POINT('Ctrl Pts',(7.56960218122422,-0.355688097435077,2.65381590527583));
#8081=CARTESIAN_POINT('Ctrl Pts',(7.69596854078112,-0.0518610909867873,
2.71393040986061));
#8082=CARTESIAN_POINT('Ctrl Pts',(7.64605614650999,0.195429699182056,2.7626228521922));
#8083=CARTESIAN_POINT('Ctrl Pts',(7.54075491725149,0.353823956190948,2.79943586318946));
#8084=CARTESIAN_POINT('Ctrl Pts',(7.38110265703664,0.460523419655934,2.83652916749481));
#8085=CARTESIAN_POINT('Ctrl Pts',(7.19162995349104,0.498419629258629,2.8738910248991));
#8086=CARTESIAN_POINT('Ctrl Pts',(7.0007409604579,0.460513246952508,2.91150596794594));
#8087=CARTESIAN_POINT('Ctrl Pts',(6.8378190554252,0.35188377722391,2.94935771811315));
#8088=CARTESIAN_POINT('Ctrl Pts',(6.72839911208997,0.188136424398707,2.98743075002918));
#8089=CARTESIAN_POINT('Ctrl Pts',(6.6852206077216,-0.027573090972768,3.02995304677867));
#8090=CARTESIAN_POINT('Ctrl Pts',(6.74868061440645,-0.266253983865906,3.07699473012916));
#8091=CARTESIAN_POINT('Ctrl Pts',(6.94034313197966,-0.457833475149794,3.12857952778403));
#8092=CARTESIAN_POINT('Ctrl Pts',(7.18108231512846,-0.522550362879875,3.17606797384646));
#8093=CARTESIAN_POINT('Ctrl Pts',(7.40075884064422,-0.478672810860648,3.21935714251314));
#8094=CARTESIAN_POINT('Ctrl Pts',(7.56869285653519,-0.36664527074508,3.25838491270649));
#8095=CARTESIAN_POINT('Ctrl Pts',(7.6809146021808,-0.198518993827375,3.29745824706686));
#8096=CARTESIAN_POINT('Ctrl Pts',(7.72493145536016,0.0218557872720809,3.34089199698168));
#8097=CARTESIAN_POINT('Ctrl Pts',(7.66010664182934,0.264194720858232,3.38867061296822));
#8098=CARTESIAN_POINT('Ctrl Pts',(7.46671346168776,0.457539735933546,3.44072387544023));
#8099=CARTESIAN_POINT('Ctrl Pts',(7.2032901519641,0.527875728031689,3.4926477940433));
#8100=CARTESIAN_POINT('Ctrl Pts',(6.94079711565823,0.457422432694776,3.54439453030441));
#8101=CARTESIAN_POINT('Ctrl Pts',(6.74965929517197,0.266025262881375,3.59590534648784));
#8102=CARTESIAN_POINT('Ctrl Pts',(6.68015786626903,0.00608630836071941,
3.64713029215759));
#8103=CARTESIAN_POINT('Ctrl Pts',(6.74970359576674,-0.251928649994077,3.69801546363488));
#8104=CARTESIAN_POINT('Ctrl Pts',(6.93743508922121,-0.439308050996682,3.74852062578755));
#8105=CARTESIAN_POINT('Ctrl Pts',(7.19159056427377,-0.50709195756326,3.79860202870109));
#8106=CARTESIAN_POINT('Ctrl Pts',(7.44320748400448,-0.439333440360368,3.84822217082346));
#8107=CARTESIAN_POINT('Ctrl Pts',(7.62546589133706,-0.256624352508281,3.89734864174091));
#8108=CARTESIAN_POINT('Ctrl Pts',(7.68558445816876,-0.0305285469163073,
3.94190287089586));
#8109=CARTESIAN_POINT('Ctrl Pts',(7.64478426817293,0.172960025251268,3.98201095418908));
#8110=CARTESIAN_POINT('Ctrl Pts',(7.5418513016088,0.326832385706015,4.01779422709743));
#8111=CARTESIAN_POINT('Ctrl Pts',(7.38915121379287,0.428586196765497,4.05326072065034));
#8112=CARTESIAN_POINT('Ctrl Pts',(7.21079763277669,0.46396249107695,4.08840353362013));
#8113=CARTESIAN_POINT('Ctrl Pts',(7.03414323162941,0.428588492367169,4.12322269578801));
#8114=CARTESIAN_POINT('Ctrl Pts',(6.88581499534645,0.32933817966448,4.15771807315783));
#8115=CARTESIAN_POINT('Ctrl Pts',(6.78768181868934,0.182230564928744,4.19189009323567));
#8116=CARTESIAN_POINT('Ctrl Pts',(6.75365398677738,0.0103830219909102,4.22574466876761));
#8117=CARTESIAN_POINT('Ctrl Pts',(6.78772267677417,-0.15978639102865,4.2592862906232));
#8118=CARTESIAN_POINT('Ctrl Pts',(6.88332961654354,-0.30275014299038,4.29252038306181));
#8119=CARTESIAN_POINT('Ctrl Pts',(7.02515283508868,-0.397267137420018,4.32545966111404));
#8120=CARTESIAN_POINT('Ctrl Pts',(7.19087475875782,-0.430188336599795,4.35811115340979));
#8121=CARTESIAN_POINT('Ctrl Pts',(7.3551529846964,-0.397308309221955,4.39049217898679));
#8122=CARTESIAN_POINT('Ctrl Pts',(7.49330452445524,-0.304979351139395,4.42260903882481));
#8123=CARTESIAN_POINT('Ctrl Pts',(7.58477684160338,-0.167677553124076,4.4544919711552));
#8124=CARTESIAN_POINT('Ctrl Pts',(7.60603157928287,-0.0607527067041877,
4.47557921241636));
#8125=CARTESIAN_POINT('Ctrl Pts',(7.60603881261167,-0.00709059188521041,
4.48612173359858));
#8126=CARTESIAN_POINT('Ctrl Pts',(7.69467762570738,0.00688377669667897,
0.514991785163569));
#8127=CARTESIAN_POINT('Ctrl Pts',(7.69466889634804,0.071643808641503,0.527714615899426));
#8128=CARTESIAN_POINT('Ctrl Pts',(7.66895523814051,0.200905554952867,0.553210400550609));
#8129=CARTESIAN_POINT('Ctrl Pts',(7.55861816964784,0.36638273901977,0.591647870327449));
#8130=CARTESIAN_POINT('Ctrl Pts',(7.39259185449073,0.477265432322967,0.630241145729233));
#8131=CARTESIAN_POINT('Ctrl Pts',(7.19606255211317,0.516492063005455,0.668976010840586));
#8132=CARTESIAN_POINT('Ctrl Pts',(6.99892977540135,0.477230860818582,0.707826422052664));
#8133=CARTESIAN_POINT('Ctrl Pts',(6.83130768528331,0.365352713499376,0.746771527227674));
#8134=CARTESIAN_POINT('Ctrl Pts',(6.71925167676417,0.197519798506761,0.785785725774557));
#8135=CARTESIAN_POINT('Ctrl Pts',(6.67963411333354,-0.000791202693221011,
0.824846572270052));
#8136=CARTESIAN_POINT('Ctrl Pts',(6.71941350175141,-0.198811372269768,0.86392807407511));
#8137=CARTESIAN_POINT('Ctrl Pts',(6.86843522759788,-0.423792949454481,0.916033400754273));
#8138=CARTESIAN_POINT('Ctrl Pts',(7.19769392010731,-0.560513248480779,0.981095150002627));
#8139=CARTESIAN_POINT('Ctrl Pts',(7.52570147928999,-0.423903016810727,1.04590305884835));
#8140=CARTESIAN_POINT('Ctrl Pts',(7.67286762063526,-0.200965968483773,1.09750364116457));
#8141=CARTESIAN_POINT('Ctrl Pts',(7.72261295254984,0.0451393462758144,1.14605420709187));
#8142=CARTESIAN_POINT('Ctrl Pts',(7.61524234685028,0.340210842305179,1.20425346675242));
#8143=CARTESIAN_POINT('Ctrl Pts',(7.29912138428851,0.52136233941282,1.27174458894949));
#8144=CARTESIAN_POINT('Ctrl Pts',(6.97463054860487,0.463557001358796,1.33292698038332));
#8145=CARTESIAN_POINT('Ctrl Pts',(6.77081821446351,0.258121233797634,1.38794832985624));
#8146=CARTESIAN_POINT('Ctrl Pts',(6.70446235354691,0.0097120224784632,1.4369679279528));
#8147=CARTESIAN_POINT('Ctrl Pts',(6.77064080749259,-0.236368179035901,1.48545948666572));
#8148=CARTESIAN_POINT('Ctrl Pts',(6.94903692491188,-0.41407503667784,1.53341005809338));
#8149=CARTESIAN_POINT('Ctrl Pts',(7.18950979304665,-0.478139101185346,1.5807967612744));
#8150=CARTESIAN_POINT('Ctrl Pts',(7.4269086887867,-0.414104038473914,1.62761310972582));
#8151=CARTESIAN_POINT('Ctrl Pts',(7.59834160025041,-0.242113962547365,1.67385370366622));
#8152=CARTESIAN_POINT('Ctrl Pts',(7.66003675045965,-0.0103513232519091,
1.7195211704181));
#8153=CARTESIAN_POINT('Ctrl Pts',(7.59836117318194,0.218336823777539,1.76462300661926));
#8154=CARTESIAN_POINT('Ctrl Pts',(7.43265726637053,0.383504832459041,1.80917303346396));
#8155=CARTESIAN_POINT('Ctrl Pts',(7.20928361949127,0.442992153199741,1.85319029170689));
#8156=CARTESIAN_POINT('Ctrl Pts',(6.98863987248015,0.38351198596622,1.89669991461219));
#8157=CARTESIAN_POINT('Ctrl Pts',(6.82910226668574,0.223518600666567,1.93973098682015));
#8158=CARTESIAN_POINT('Ctrl Pts',(6.77139704108765,0.00734290766390798,
1.98232025113029));
#8159=CARTESIAN_POINT('Ctrl Pts',(6.81955140322323,-0.17080763583515,2.01747249154634));
#8160=CARTESIAN_POINT('Ctrl Pts',(6.90677940492032,-0.284130764144419,2.0454129068512));
#8161=CARTESIAN_POINT('Ctrl Pts',(7.01970141686137,-0.370956746763405,2.07324122060183));
#8162=CARTESIAN_POINT('Ctrl Pts',(7.19517285585778,-0.417865627882994,2.10783440889197));
#8163=CARTESIAN_POINT('Ctrl Pts',(7.40439082299913,-0.361726044210867,2.14907886919864));
#8164=CARTESIAN_POINT('Ctrl Pts',(7.55671510006043,-0.209184076105135,2.19011719492698));
#8165=CARTESIAN_POINT('Ctrl Pts',(7.60748456033901,-0.0190531027858145,
2.22759299177402));
#8166=CARTESIAN_POINT('Ctrl Pts',(7.57300852841629,0.153433881101946,2.26158938023144));
#8167=CARTESIAN_POINT('Ctrl Pts',(7.48522152825439,0.284973433685168,2.29215525097081));
#8168=CARTESIAN_POINT('Ctrl Pts',(7.35371479002735,0.37272858905955,2.32271540904616));
#8169=CARTESIAN_POINT('Ctrl Pts',(7.18132429762203,0.407224317027577,2.35669104556836));
#8170=CARTESIAN_POINT('Ctrl Pts',(6.9913809597726,0.356397258300469,2.39412528364257));
#8171=CARTESIAN_POINT('Ctrl Pts',(6.83922114282842,0.204287390367652,2.43509680013667));
#8172=CARTESIAN_POINT('Ctrl Pts',(6.78776554029098,0.0128275311884052,2.47282559318833));
#8173=CARTESIAN_POINT('Ctrl Pts',(6.82279513668012,-0.161901812992041,2.50730303808298));
#8174=CARTESIAN_POINT('Ctrl Pts',(6.94158088523551,-0.34159342973453,2.54888699780782));
#8175=CARTESIAN_POINT('Ctrl Pts',(7.20629039228909,-0.452427791333231,2.60131567268228));
#8176=CARTESIAN_POINT('Ctrl Pts',(7.5304300988666,-0.319328872462905,2.66510484392403));
#8177=CARTESIAN_POINT('Ctrl Pts',(7.64393545484647,-0.0463609609462171,
2.71910010788248));
#8178=CARTESIAN_POINT('Ctrl Pts',(7.59909834565696,0.175907590184711,2.76286026063545));
#8179=CARTESIAN_POINT('Ctrl Pts',(7.50438991288635,0.318409515321193,2.79597016810716));
#8180=CARTESIAN_POINT('Ctrl Pts',(7.3605799039455,0.414556437496516,2.82938176955588));
#8181=CARTESIAN_POINT('Ctrl Pts',(7.18955265969801,0.448811059922502,2.86310195270141));
#8182=CARTESIAN_POINT('Ctrl Pts',(7.01678655931437,0.414550262799124,2.89713771190015));
#8183=CARTESIAN_POINT('Ctrl Pts',(6.86885174085118,0.315990474399967,2.93149384807802));
#8184=CARTESIAN_POINT('Ctrl Pts',(6.76911069802026,0.166845046570867,2.96617128633524));
#8185=CARTESIAN_POINT('Ctrl Pts',(6.72953139858562,-0.0304522148375183,
3.00506495776769));
#8186=CARTESIAN_POINT('Ctrl Pts',(6.78769390474188,-0.249937774164215,3.04830039529776));
#8187=CARTESIAN_POINT('Ctrl Pts',(6.9649370626522,-0.427422514214055,3.09603683868771));
#8188=CARTESIAN_POINT('Ctrl Pts',(7.18932018203905,-0.487979620328074,3.14030064536012));
#8189=CARTESIAN_POINT('Ctrl Pts',(7.39557279768717,-0.446904315163521,3.18093085548355));
#8190=CARTESIAN_POINT('Ctrl Pts',(7.55425360364287,-0.341191109504664,3.21778878121054));
#8191=CARTESIAN_POINT('Ctrl Pts',(7.66102690207568,-0.181435475111084,3.25492379188564));
#8192=CARTESIAN_POINT('Ctrl Pts',(7.70328741298565,0.0294016985791167,3.2964816011759));
#8193=CARTESIAN_POINT('Ctrl Pts',(7.64104047721324,0.263177246401401,3.34254524203817));
#8194=CARTESIAN_POINT('Ctrl Pts',(7.45302343605178,0.451617524859523,3.39320364580977));
#8195=CARTESIAN_POINT('Ctrl Pts',(7.19421186989991,0.521059884552374,3.44422754118507));
#8196=CARTESIAN_POINT('Ctrl Pts',(6.93366759288141,0.451480374799088,3.49556420787452));
#8197=CARTESIAN_POINT('Ctrl Pts',(6.74192572911501,0.259952952462136,3.54716607559634));
#8198=CARTESIAN_POINT('Ctrl Pts',(6.67128705932614,-0.00291987582538055,
3.59897914569118));
#8199=CARTESIAN_POINT('Ctrl Pts',(6.74200130890162,-0.266556153752997,3.65095085469123));
#8200=CARTESIAN_POINT('Ctrl Pts',(6.93533270564664,-0.459989954442243,3.70302170351135));
#8201=CARTESIAN_POINT('Ctrl Pts',(7.19973042361935,-0.530836528881026,3.75513473434544));
#8202=CARTESIAN_POINT('Ctrl Pts',(7.46399256228725,-0.459988881699339,3.80723200840435));
#8203=CARTESIAN_POINT('Ctrl Pts',(7.65720752588036,-0.266714233190792,3.85925510262137));
#8204=CARTESIAN_POINT('Ctrl Pts',(7.72162850029991,-0.0253919365293239,
3.90682319346266));
#8205=CARTESIAN_POINT('Ctrl Pts',(7.67789482230646,0.193331762568851,3.94992933060867));
#8206=CARTESIAN_POINT('Ctrl Pts',(7.56675267456708,0.359645580693078,3.98859787225562));
#8207=CARTESIAN_POINT('Ctrl Pts',(7.40097626920353,0.47022490567555,4.02711395823539));
#8208=CARTESIAN_POINT('Ctrl Pts',(7.20640719990281,0.508899267550811,4.06545972626007));
#8209=CARTESIAN_POINT('Ctrl Pts',(7.01283946983003,0.470213246623792,4.1036131517629));
#8210=CARTESIAN_POINT('Ctrl Pts',(6.84967688295545,0.36111126628715,4.1415548777527));
#8211=CARTESIAN_POINT('Ctrl Pts',(6.74134731945609,0.198812605531192,4.17926855876961));
#8212=CARTESIAN_POINT('Ctrl Pts',(6.70365533298111,0.00866379922224738,
4.21673517440635));
#8213=CARTESIAN_POINT('Ctrl Pts',(6.74140931659415,-0.180078545667991,4.25394103083648));
#8214=CARTESIAN_POINT('Ctrl Pts',(6.84762388733812,-0.338921159861923,4.29087272651501));
#8215=CARTESIAN_POINT('Ctrl Pts',(7.00537067407869,-0.444065320510892,4.3275172120746));
#8216=CARTESIAN_POINT('Ctrl Pts',(7.18981724442161,-0.480695590575098,4.36386348999543));
#8217=CARTESIAN_POINT('Ctrl Pts',(7.37263926416229,-0.444099896756117,4.399905298103));
#8218=CARTESIAN_POINT('Ctrl Pts',(7.52627543630935,-0.341400177175117,4.43562905755834));
#8219=CARTESIAN_POINT('Ctrl Pts',(7.62785720298341,-0.188901379750348,4.47104576944789));
#8220=CARTESIAN_POINT('Ctrl Pts',(7.65140397112763,-0.0703858575854634,
4.49442272113103));
#8221=CARTESIAN_POINT('Ctrl Pts',(7.6514119734328,-0.0110189146175235,4.50608601945378));
#8222=CARTESIAN_POINT('Ctrl Pts',(7.66495866561397,0.0096408208356154,0.500937861339137));
#8223=CARTESIAN_POINT('Ctrl Pts',(7.66495043542855,0.0706976578322391,0.512933158114727));
#8224=CARTESIAN_POINT('Ctrl Pts',(7.6407288414539,0.192578461749219,0.53697092906723));
#8225=CARTESIAN_POINT('Ctrl Pts',(7.53641483655384,0.349135128226674,0.57332721437664));
#8226=CARTESIAN_POINT('Ctrl Pts',(7.37891862529407,0.454388959539344,0.609942269987145));
#8227=CARTESIAN_POINT('Ctrl Pts',(7.19182916610252,0.491804928705749,0.646817568764298));
#8228=CARTESIAN_POINT('Ctrl Pts',(7.00345300936995,0.454364611540757,0.683937116394234));
#8229=CARTESIAN_POINT('Ctrl Pts',(6.8426331207003,0.347126595132945,0.72128862247113));
#8230=CARTESIAN_POINT('Ctrl Pts',(6.73465279105392,0.185548007545082,0.758857805369577));
#8231=CARTESIAN_POINT('Ctrl Pts',(6.69624812122046,-0.00620356043593041,
0.796628033574345));
#8232=CARTESIAN_POINT('Ctrl Pts',(6.73480718344848,-0.198554484110674,0.834582940724046));
#8233=CARTESIAN_POINT('Ctrl Pts',(6.88005293713107,-0.418084886861934,0.885411952478362));
#8234=CARTESIAN_POINT('Ctrl Pts',(7.20322101675746,-0.552973672355533,0.949310201794791));
#8235=CARTESIAN_POINT('Ctrl Pts',(7.52875135792009,-0.418120197994963,1.01356942995885));
#8236=CARTESIAN_POINT('Ctrl Pts',(7.67590748900772,-0.195467714230404,1.06510280128326));
#8237=CARTESIAN_POINT('Ctrl Pts',(7.72594697491113,0.051510497628374,1.11382936475781));
#8238=CARTESIAN_POINT('Ctrl Pts',(7.61792973454696,0.34980833854487,1.17261054327264));
#8239=CARTESIAN_POINT('Ctrl Pts',(7.29600845579134,0.534934534966306,1.24137836329612));
#8240=CARTESIAN_POINT('Ctrl Pts',(6.9624343826518,0.475986238152519,1.30425389372148));
#8241=CARTESIAN_POINT('Ctrl Pts',(6.7513269732076,0.263559075549507,1.36117052033831));
#8242=CARTESIAN_POINT('Ctrl Pts',(6.68208673935486,0.00506624913794415,
1.41217539507843));
#8243=CARTESIAN_POINT('Ctrl Pts',(6.75115729338842,-0.252515030784761,1.46291637360071));
#8244=CARTESIAN_POINT('Ctrl Pts',(6.93868139789632,-0.439549141627597,1.51333206514984));
#8245=CARTESIAN_POINT('Ctrl Pts',(7.19277218532913,-0.507400915671182,1.56339686963768));
#8246=CARTESIAN_POINT('Ctrl Pts',(7.44475704014889,-0.439568775677871,1.6130666625822));
#8247=CARTESIAN_POINT('Ctrl Pts',(7.62746056234528,-0.256432683273915,1.66231123683637));
#8248=CARTESIAN_POINT('Ctrl Pts',(7.69348210450095,-0.00877779198086032,
1.71110033955553));
#8249=CARTESIAN_POINT('Ctrl Pts',(7.62746910095865,0.236264427972525,1.75941038595882));
#8250=CARTESIAN_POINT('Ctrl Pts',(7.44962012238075,0.413605394268341,1.80722176291839));
#8251=CARTESIAN_POINT('Ctrl Pts',(7.20954044812925,0.477565743583523,1.85452048529808));
#8252=CARTESIAN_POINT('Ctrl Pts',(6.97227231959396,0.413602123353752,1.90129735375243));
#8253=CARTESIAN_POINT('Ctrl Pts',(6.80077909361189,0.241579533289261,1.94754921821389));
#8254=CARTESIAN_POINT('Ctrl Pts',(6.7388618673047,0.00940863316150851,1.9932768407136));
#8255=CARTESIAN_POINT('Ctrl Pts',(6.79054491525727,-0.181541982999997,2.03095403885583));
#8256=CARTESIAN_POINT('Ctrl Pts',(6.88387815366437,-0.302767035565214,2.06084460346816));
#8257=CARTESIAN_POINT('Ctrl Pts',(7.00451694241951,-0.395503980057399,2.09056986286438));
#8258=CARTESIAN_POINT('Ctrl Pts',(7.19149482154426,-0.445378090698615,2.1274222004115));
#8259=CARTESIAN_POINT('Ctrl Pts',(7.41343391189553,-0.385678179322762,2.17118156013989));
#8260=CARTESIAN_POINT('Ctrl Pts',(7.57412088328951,-0.224511384987361,2.21450495485577));
#8261=CARTESIAN_POINT('Ctrl Pts',(7.62724779211325,-0.0248721738545197,
2.25384933801546));
#8262=CARTESIAN_POINT('Ctrl Pts',(7.59116361468395,0.155190246720775,2.28934298364047));
#8263=CARTESIAN_POINT('Ctrl Pts',(7.49989052392447,0.291790939188551,2.32109884315156));
#8264=CARTESIAN_POINT('Ctrl Pts',(7.36395007742405,0.38239718016914,2.35268032633859));
#8265=CARTESIAN_POINT('Ctrl Pts',(7.18676166604564,0.417742312375305,2.38759960338815));
#8266=CARTESIAN_POINT('Ctrl Pts',(6.99291266772421,0.365648667519335,2.42582318365208));
#8267=CARTESIAN_POINT('Ctrl Pts',(6.83897107184478,0.211431047408248,2.46732314866766));
#8268=CARTESIAN_POINT('Ctrl Pts',(6.78748883973987,0.0190035426787835,2.50524603217002));
#8269=CARTESIAN_POINT('Ctrl Pts',(6.82252928042011,-0.155278930965659,2.53965006117662));
#8270=CARTESIAN_POINT('Ctrl Pts',(6.94047269326526,-0.333425126549853,2.58089918196454));
#8271=CARTESIAN_POINT('Ctrl Pts',(7.20090707643882,-0.441779652078452,2.63244776860263));
#8272=CARTESIAN_POINT('Ctrl Pts',(7.51563071205169,-0.311721566968956,2.69446142088775));
#8273=CARTESIAN_POINT('Ctrl Pts',(7.62430311252255,-0.0489647930063533,
2.74642328448686));
#8274=CARTESIAN_POINT('Ctrl Pts',(7.5813840421979,0.163308287319331,2.78823405894546));
#8275=CARTESIAN_POINT('Ctrl Pts',(7.49123285044309,0.298833086231118,2.81973896360247));
#8276=CARTESIAN_POINT('Ctrl Pts',(7.35493116122275,0.389891719124265,2.85140756747005));
#8277=CARTESIAN_POINT('Ctrl Pts',(7.19341536220524,0.422180171213018,2.88325853512063));
#8278=CARTESIAN_POINT('Ctrl Pts',(7.03077842930683,0.389887859695428,2.91530957463356));
#8279=CARTESIAN_POINT('Ctrl Pts',(6.89190449463321,0.297309810814242,2.94757450110591));
#8280=CARTESIAN_POINT('Ctrl Pts',(6.79848642055615,0.157571536298674,2.98007238787189));
#8281=CARTESIAN_POINT('Ctrl Pts',(6.76150685487504,-0.0269250762532582,
3.01644525951301));
#8282=CARTESIAN_POINT('Ctrl Pts',(6.81585071674324,-0.231845001847761,3.05683113794882));
#8283=CARTESIAN_POINT('Ctrl Pts',(6.98114939225645,-0.397360174681789,3.101361111042));
#8284=CARTESIAN_POINT('Ctrl Pts',(7.19033341376853,-0.453815928881707,3.14263718537585));
#8285=CARTESIAN_POINT('Ctrl Pts',(7.38267033377326,-0.415535666902471,3.18053365000396));
#8286=CARTESIAN_POINT('Ctrl Pts',(7.5307464143918,-0.316904538681263,3.21493081649486));
#8287=CARTESIAN_POINT('Ctrl Pts',(7.63050738643256,-0.167696568139501,3.24962471887291));
#8288=CARTESIAN_POINT('Ctrl Pts',(7.67006526296691,0.0295052786481756,3.28849853708803));
#8289=CARTESIAN_POINT('Ctrl Pts',(7.61180808226649,0.248648829409802,3.3316858887866));
#8290=CARTESIAN_POINT('Ctrl Pts',(7.43514984947071,0.425869407836813,3.37931317995539));
#8291=CARTESIAN_POINT('Ctrl Pts',(7.19106330905834,0.491496622933082,3.42744471708512));
#8292=CARTESIAN_POINT('Ctrl Pts',(6.94429664016134,0.425752312282669,3.47606216769791));
#8293=CARTESIAN_POINT('Ctrl Pts',(6.76180911767831,0.243701545752318,3.52514523794754));
#8294=CARTESIAN_POINT('Ctrl Pts',(6.69412136518916,-0.00747982371833415,
3.57466354176041));
#8295=CARTESIAN_POINT('Ctrl Pts',(6.76187382592234,-0.260799521439724,3.62459127426534));
#8296=CARTESIAN_POINT('Ctrl Pts',(6.94847611579586,-0.447791932889458,3.67488482395855));
#8297=CARTESIAN_POINT('Ctrl Pts',(7.20529145918771,-0.516830252602251,3.72550931504893));
#8298=CARTESIAN_POINT('Ctrl Pts',(7.46363123050322,-0.447802422833225,3.77642000140872));
#8299=CARTESIAN_POINT('Ctrl Pts',(7.6538074437744,-0.257897177129994,3.82757293127415));
#8300=CARTESIAN_POINT('Ctrl Pts',(7.7177715912926,-0.0191264507767671,3.8746366938418));
#8301=CARTESIAN_POINT('Ctrl Pts',(7.67435473390573,0.198582385366778,3.91753173887265));
#8302=CARTESIAN_POINT('Ctrl Pts',(7.56329681060452,0.364957935365554,3.95619050975397));
#8303=CARTESIAN_POINT('Ctrl Pts',(7.39675108803321,0.476165093095772,3.99489365541533));
#8304=CARTESIAN_POINT('Ctrl Pts',(7.20029814145452,0.515321267550363,4.03360638733665));
#8305=CARTESIAN_POINT('Ctrl Pts',(7.00387047286649,0.476163919411364,4.07231102869526));
#8306=CARTESIAN_POINT('Ctrl Pts',(6.83746567537909,0.365016133595194,4.11098698220102));
#8307=CARTESIAN_POINT('Ctrl Pts',(6.72642378886519,0.198833317396287,4.14960586405847));
#8308=CARTESIAN_POINT('Ctrl Pts',(6.68753839413938,0.00317933679133277,
4.18815341806877));
#8309=CARTESIAN_POINT('Ctrl Pts',(6.72647710351975,-0.191933239252609,4.22660331585192));
#8310=CARTESIAN_POINT('Ctrl Pts',(6.83665572362076,-0.356887001441586,4.2649335303692));
#8311=CARTESIAN_POINT('Ctrl Pts',(7.00106911490509,-0.466565590640207,4.30312749646998));
#8312=CARTESIAN_POINT('Ctrl Pts',(7.19410690234209,-0.504987935840618,4.34116313228386));
#8313=CARTESIAN_POINT('Ctrl Pts',(7.38621803807239,-0.466593360436696,4.37902453826879));
#8314=CARTESIAN_POINT('Ctrl Pts',(7.54825768185721,-0.3583357834793,4.4166899096587));
#8315=CARTESIAN_POINT('Ctrl Pts',(7.65577203010817,-0.197002467064972,4.4541521298834));
#8316=CARTESIAN_POINT('Ctrl Pts',(7.6807779728439,-0.0711713717257019,4.47896571871842));
#8317=CARTESIAN_POINT('Ctrl Pts',(7.68078647070003,-0.00812806991155192,
4.49135127875486));
#8318=CARTESIAN_POINT('Ctrl Pts',(7.64999870073278,0.00963880430002493,
0.500937861339137));
#8319=CARTESIAN_POINT('Ctrl Pts',(7.64999072283273,0.0688240253405825,0.512565458280486));
#8320=CARTESIAN_POINT('Ctrl Pts',(7.62651906829351,0.186933280416436,0.535860737255745));
#8321=CARTESIAN_POINT('Ctrl Pts',(7.52538952050926,0.338721501716328,0.571111621876026));
#8322=CARTESIAN_POINT('Ctrl Pts',(7.37261016576107,0.440828782725881,0.606632113855559));
#8323=CARTESIAN_POINT('Ctrl Pts',(7.19098801918939,0.477160089388571,0.642432691908446));
#8324=CARTESIAN_POINT('Ctrl Pts',(7.00794887133667,0.440792445335284,0.678501299793522));
#8325=CARTESIAN_POINT('Ctrl Pts',(6.85151949944076,0.336499171833787,0.714833893830788));
#8326=CARTESIAN_POINT('Ctrl Pts',(6.74635289761356,0.179164878106423,0.751420068859459));
#8327=CARTESIAN_POINT('Ctrl Pts',(6.7088855037237,-0.00779582609077112,
0.78825059826266));
#8328=CARTESIAN_POINT('Ctrl Pts',(6.74651391108833,-0.195622387289353,0.825313313466632));
#8329=CARTESIAN_POINT('Ctrl Pts',(6.88851119015049,-0.410310488976418,0.875022999496246));
#8330=CARTESIAN_POINT('Ctrl Pts',(7.20522985356176,-0.542753193552164,0.937673401670968));
#8331=CARTESIAN_POINT('Ctrl Pts',(7.52560124560565,-0.410308950963103,1.00090311405878));
#8332=CARTESIAN_POINT('Ctrl Pts',(7.67086762315913,-0.190619832396083,1.0517623380234));
#8333=CARTESIAN_POINT('Ctrl Pts',(7.72038428103372,0.053554354178951,1.09994516441643));
#8334=CARTESIAN_POINT('Ctrl Pts',(7.61346157902179,0.349425527858921,1.15825605943124));
#8335=CARTESIAN_POINT('Ctrl Pts',(7.293147036645,0.533923363778534,1.22671892603372));
#8336=CARTESIAN_POINT('Ctrl Pts',(6.9598052915743,0.475238618295502,1.28954716027338));
#8337=CARTESIAN_POINT('Ctrl Pts',(6.74803078150055,0.262318163018047,1.34663189357301));
#8338=CARTESIAN_POINT('Ctrl Pts',(6.67830810206772,0.0023988076890563,1.3979329504908));
#8339=CARTESIAN_POINT('Ctrl Pts',(6.74786353789082,-0.257385664114871,1.44910892564238));
#8340=CARTESIAN_POINT('Ctrl Pts',(6.93745136291826,-0.446625861944449,1.50011118169226));
#8341=CARTESIAN_POINT('Ctrl Pts',(7.19511270617401,-0.515530236866011,1.55089291586215));
#8342=CARTESIAN_POINT('Ctrl Pts',(7.45136837615866,-0.446648689171563,1.60140954707133));
#8343=CARTESIAN_POINT('Ctrl Pts',(7.63768442718454,-0.260018056286165,1.65161922462518));
#8344=CARTESIAN_POINT('Ctrl Pts',(7.70523033687804,-0.0069714683683192,
1.70148323387221));
#8345=CARTESIAN_POINT('Ctrl Pts',(7.63769895751989,0.244003419049979,1.75096640161628));
#8346=CARTESIAN_POINT('Ctrl Pts',(7.45523859330254,0.426040600914326,1.80003745460796));
#8347=CARTESIAN_POINT('Ctrl Pts',(7.20843773134158,0.491855409637758,1.84866933496872));
#8348=CARTESIAN_POINT('Ctrl Pts',(6.96411419073211,0.426044527968114,1.89683949153479));
#8349=CARTESIAN_POINT('Ctrl Pts',(6.7872702247347,0.248717255937941,1.94453007704133));
#8350=CARTESIAN_POINT('Ctrl Pts',(6.72333142706999,0.00910740273079913,
1.99172820696913));
#8351=CARTESIAN_POINT('Ctrl Pts',(6.77669190792476,-0.188112629887261,2.03064296753181));
#8352=CARTESIAN_POINT('Ctrl Pts',(6.87311288530633,-0.313353108724919,2.06152326719269));
#8353=CARTESIAN_POINT('Ctrl Pts',(6.9977575234091,-0.409174440391491,2.0922362142172));
#8354=CARTESIAN_POINT('Ctrl Pts',(7.19095586866206,-0.460713817161615,2.13031448846159));
#8355=CARTESIAN_POINT('Ctrl Pts',(7.42021304552618,-0.399036009194613,2.17551521533059));
#8356=CARTESIAN_POINT('Ctrl Pts',(7.58607675038944,-0.232652998639623,2.22023530187249));
#8357=CARTESIAN_POINT('Ctrl Pts',(7.64084113722653,-0.0267711157317457,
2.2608041635776));
#8358=CARTESIAN_POINT('Ctrl Pts',(7.60365245023964,0.158696418911201,2.2973634945418));
#8359=CARTESIAN_POINT('Ctrl Pts',(7.50973838584388,0.299219822341778,2.33003006433835));
#8360=CARTESIAN_POINT('Ctrl Pts',(7.37007100234203,0.392281683236922,2.36247215334549));
#8361=CARTESIAN_POINT('Ctrl Pts',(7.18832364110351,0.428509871500047,2.39828479951764));
#8362=CARTESIAN_POINT('Ctrl Pts',(6.98993152312495,0.375130255900093,2.43739940337039));
#8363=CARTESIAN_POINT('Ctrl Pts',(6.83283942785452,0.217642962930976,2.47976008769737));
#8364=CARTESIAN_POINT('Ctrl Pts',(6.7805179762894,0.0217759129571612,2.51834494637949));
#8365=CARTESIAN_POINT('Ctrl Pts',(6.81611962546049,-0.155110783437508,2.55325894844757));
#8366=CARTESIAN_POINT('Ctrl Pts',(6.93559514558806,-0.335467183812974,2.59501419582854));
#8367=CARTESIAN_POINT('Ctrl Pts',(7.19838636703693,-0.444497554803198,2.64699296075227));
#8368=CARTESIAN_POINT('Ctrl Pts',(7.51396784981042,-0.313675439428632,2.70919005501935));
#8369=CARTESIAN_POINT('Ctrl Pts',(7.62212313812957,-0.0514208051434247,
2.76101600110827));
#8370=CARTESIAN_POINT('Ctrl Pts',(7.57941022831611,0.159498854704775,2.80255943176652));
#8371=CARTESIAN_POINT('Ctrl Pts',(7.49002790476542,0.293811387305209,2.83377939972915));
#8372=CARTESIAN_POINT('Ctrl Pts',(7.3552499441484,0.383795703607156,2.86508254302445));
#8373=CARTESIAN_POINT('Ctrl Pts',(7.19595280633545,0.41560735445773,2.89648910888395));
#8374=CARTESIAN_POINT('Ctrl Pts',(7.03593949389396,0.383792650446306,2.92801879141503));
#8375=CARTESIAN_POINT('Ctrl Pts',(6.89961651509014,0.292876470296345,2.95969053299985));
#8376=CARTESIAN_POINT('Ctrl Pts',(6.8081238548802,0.155952445855146,2.99152250722056));
#8377=CARTESIAN_POINT('Ctrl Pts',(6.7719951154116,-0.0244720795860329,3.02708849903104));
#8378=CARTESIAN_POINT('Ctrl Pts',(6.82508694038131,-0.224423780156864,3.0664872528009));
#8379=CARTESIAN_POINT('Ctrl Pts',(6.9861130399098,-0.385566648672682,3.1098474493302));
#8380=CARTESIAN_POINT('Ctrl Pts',(7.18949761386412,-0.440411898981026,3.14997109794484));
#8381=CARTESIAN_POINT('Ctrl Pts',(7.37626527013998,-0.403213775048244,3.18676673081186));
#8382=CARTESIAN_POINT('Ctrl Pts',(7.51993103796524,-0.30750405465344,3.2201390303787));
#8383=CARTESIAN_POINT('Ctrl Pts',(7.61665044076158,-0.16281791922389,3.25377599756719));
#8384=CARTESIAN_POINT('Ctrl Pts',(7.65498225700094,0.0283123086785322,3.29145196922942));
#8385=CARTESIAN_POINT('Ctrl Pts',(7.59852316170633,0.240631420079613,3.3332902111484));
#8386=CARTESIAN_POINT('Ctrl Pts',(7.42736589163809,0.412328652603764,3.37943210760514));
#8387=CARTESIAN_POINT('Ctrl Pts',(7.19081184831391,0.475941162716025,3.42607713455886));
#8388=CARTESIAN_POINT('Ctrl Pts',(6.95151342469985,0.412204069493947,3.47322302929114));
#8389=CARTESIAN_POINT('Ctrl Pts',(6.77437422620912,0.235528496642651,3.52086247665056));
#8390=CARTESIAN_POINT('Ctrl Pts',(6.70856719057301,-0.00853695568196444,
3.56898306053165));
#8391=CARTESIAN_POINT('Ctrl Pts',(6.77444746404088,-0.255049338492359,3.61756749823055));
#8392=CARTESIAN_POINT('Ctrl Pts',(6.9562898685306,-0.437346140614658,3.66659366870206));
#8393=CARTESIAN_POINT('Ctrl Pts',(7.20705837195632,-0.504822359013845,3.71603499825878));
#8394=CARTESIAN_POINT('Ctrl Pts',(7.45987118758895,-0.437340247483335,3.76586064283255));
#8395=CARTESIAN_POINT('Ctrl Pts',(7.64643847266503,-0.251145802482984,3.81603581337119));
#8396=CARTESIAN_POINT('Ctrl Pts',(7.70939130979041,-0.0164226811455054,
3.86231497498143));
#8397=CARTESIAN_POINT('Ctrl Pts',(7.66665300702434,0.198091300428752,3.90458351454994));
#8398=CARTESIAN_POINT('Ctrl Pts',(7.55703831361006,0.362363180751678,3.94275824199772));
#8399=CARTESIAN_POINT('Ctrl Pts',(7.39231161872226,0.472405147713809,3.98104671473859));
#8400=CARTESIAN_POINT('Ctrl Pts',(7.19757748614764,0.511253819560404,4.01942894411337));
#8401=CARTESIAN_POINT('Ctrl Pts',(7.00243742159468,0.472394913482402,4.05788442705078));
#8402=CARTESIAN_POINT('Ctrl Pts',(6.83675859423202,0.361776141956741,4.09639221672569));
#8403=CARTESIAN_POINT('Ctrl Pts',(6.72593678453896,0.195994806221917,4.13493108529455));
#8404=CARTESIAN_POINT('Ctrl Pts',(6.6870196897812,0.000372767277272366,
4.17347960299015));
#8405=CARTESIAN_POINT('Ctrl Pts',(6.72599808190112,-0.19515902350661,4.21201632288769));
#8406=CARTESIAN_POINT('Ctrl Pts',(6.83662574734572,-0.360840864201945,4.25051978478148));
#8407=CARTESIAN_POINT('Ctrl Pts',(7.00208504736442,-0.47127212461887,4.28896891774833));
#8408=CARTESIAN_POINT('Ctrl Pts',(7.19679737636779,-0.510060779189973,4.32734248506513));
#8409=CARTESIAN_POINT('Ctrl Pts',(7.39100313831524,-0.471299286801184,4.36562087591661));
#8410=CARTESIAN_POINT('Ctrl Pts',(7.5551719819179,-0.361667391724164,4.40378216412631));
#8411=CARTESIAN_POINT('Ctrl Pts',(7.66435033350436,-0.197951056928272,4.44181269280615));
#8412=CARTESIAN_POINT('Ctrl Pts',(7.68982126235038,-0.0699660743691742,
4.46705762798012));
#8413=CARTESIAN_POINT('Ctrl Pts',(7.68982990724746,-0.00583191542195246,
4.4796574990714));
#8414=CARTESIAN_POINT('',(7.64999870073278,0.00963880430002493,0.500937861339137));
#8415=CARTESIAN_POINT('Origin',(7.65,-1.95245324213388E-18,0.55));
#8416=CARTESIAN_POINT('',(7.68982990724746,-0.00583191542195245,4.4796574990714));
#8417=CARTESIAN_POINT('Ctrl Pts',(7.64999870073278,0.00963880430002493,
0.500937861339137));
#8418=CARTESIAN_POINT('Ctrl Pts',(7.64999072283273,0.0688240253405825,0.512565458280486));
#8419=CARTESIAN_POINT('Ctrl Pts',(7.62651906829351,0.186933280416436,0.535860737255745));
#8420=CARTESIAN_POINT('Ctrl Pts',(7.52538952050926,0.338721501716328,0.571111621876026));
#8421=CARTESIAN_POINT('Ctrl Pts',(7.37261016576107,0.440828782725881,0.606632113855559));
#8422=CARTESIAN_POINT('Ctrl Pts',(7.19098801918939,0.477160089388571,0.642432691908446));
#8423=CARTESIAN_POINT('Ctrl Pts',(7.00794887133667,0.440792445335284,0.678501299793522));
#8424=CARTESIAN_POINT('Ctrl Pts',(6.85151949944076,0.336499171833787,0.714833893830788));
#8425=CARTESIAN_POINT('Ctrl Pts',(6.74635289761356,0.179164878106423,0.751420068859459));
#8426=CARTESIAN_POINT('Ctrl Pts',(6.7088855037237,-0.00779582609077112,
0.78825059826266));
#8427=CARTESIAN_POINT('Ctrl Pts',(6.74651391108833,-0.195622387289353,0.825313313466632));
#8428=CARTESIAN_POINT('Ctrl Pts',(6.88851119015049,-0.410310488976418,0.875022999496246));
#8429=CARTESIAN_POINT('Ctrl Pts',(7.20522985356176,-0.542753193552164,0.937673401670968));
#8430=CARTESIAN_POINT('Ctrl Pts',(7.52560124560565,-0.410308950963103,1.00090311405878));
#8431=CARTESIAN_POINT('Ctrl Pts',(7.67086762315913,-0.190619832396083,1.0517623380234));
#8432=CARTESIAN_POINT('Ctrl Pts',(7.72038428103372,0.053554354178951,1.09994516441643));
#8433=CARTESIAN_POINT('Ctrl Pts',(7.61346157902179,0.349425527858921,1.15825605943124));
#8434=CARTESIAN_POINT('Ctrl Pts',(7.293147036645,0.533923363778534,1.22671892603372));
#8435=CARTESIAN_POINT('Ctrl Pts',(6.9598052915743,0.475238618295502,1.28954716027338));
#8436=CARTESIAN_POINT('Ctrl Pts',(6.74803078150055,0.262318163018047,1.34663189357301));
#8437=CARTESIAN_POINT('Ctrl Pts',(6.67830810206772,0.0023988076890563,1.3979329504908));
#8438=CARTESIAN_POINT('Ctrl Pts',(6.74786353789082,-0.257385664114871,1.44910892564238));
#8439=CARTESIAN_POINT('Ctrl Pts',(6.93745136291826,-0.446625861944449,1.50011118169226));
#8440=CARTESIAN_POINT('Ctrl Pts',(7.19511270617401,-0.515530236866011,1.55089291586215));
#8441=CARTESIAN_POINT('Ctrl Pts',(7.45136837615866,-0.446648689171563,1.60140954707133));
#8442=CARTESIAN_POINT('Ctrl Pts',(7.63768442718454,-0.260018056286165,1.65161922462518));
#8443=CARTESIAN_POINT('Ctrl Pts',(7.70523033687804,-0.0069714683683192,
1.70148323387221));
#8444=CARTESIAN_POINT('Ctrl Pts',(7.63769895751989,0.244003419049979,1.75096640161628));
#8445=CARTESIAN_POINT('Ctrl Pts',(7.45523859330254,0.426040600914326,1.80003745460796));
#8446=CARTESIAN_POINT('Ctrl Pts',(7.20843773134158,0.491855409637758,1.84866933496872));
#8447=CARTESIAN_POINT('Ctrl Pts',(6.96411419073211,0.426044527968114,1.89683949153479));
#8448=CARTESIAN_POINT('Ctrl Pts',(6.7872702247347,0.248717255937941,1.94453007704133));
#8449=CARTESIAN_POINT('Ctrl Pts',(6.72333142706999,0.00910740273079913,
1.99172820696913));
#8450=CARTESIAN_POINT('Ctrl Pts',(6.77669190792476,-0.188112629887261,2.03064296753181));
#8451=CARTESIAN_POINT('Ctrl Pts',(6.87311288530633,-0.313353108724919,2.06152326719269));
#8452=CARTESIAN_POINT('Ctrl Pts',(6.9977575234091,-0.409174440391491,2.0922362142172));
#8453=CARTESIAN_POINT('Ctrl Pts',(7.19095586866206,-0.460713817161615,2.13031448846159));
#8454=CARTESIAN_POINT('Ctrl Pts',(7.42021304552618,-0.399036009194613,2.17551521533059));
#8455=CARTESIAN_POINT('Ctrl Pts',(7.58607675038944,-0.232652998639623,2.22023530187249));
#8456=CARTESIAN_POINT('Ctrl Pts',(7.64084113722653,-0.0267711157317457,
2.2608041635776));
#8457=CARTESIAN_POINT('Ctrl Pts',(7.60365245023964,0.158696418911201,2.2973634945418));
#8458=CARTESIAN_POINT('Ctrl Pts',(7.50973838584388,0.299219822341778,2.33003006433835));
#8459=CARTESIAN_POINT('Ctrl Pts',(7.37007100234203,0.392281683236922,2.36247215334549));
#8460=CARTESIAN_POINT('Ctrl Pts',(7.18832364110351,0.428509871500047,2.39828479951764));
#8461=CARTESIAN_POINT('Ctrl Pts',(6.98993152312495,0.375130255900093,2.43739940337039));
#8462=CARTESIAN_POINT('Ctrl Pts',(6.83283942785452,0.217642962930976,2.47976008769737));
#8463=CARTESIAN_POINT('Ctrl Pts',(6.7805179762894,0.0217759129571612,2.51834494637949));
#8464=CARTESIAN_POINT('Ctrl Pts',(6.81611962546049,-0.155110783437508,2.55325894844757));
#8465=CARTESIAN_POINT('Ctrl Pts',(6.93559514558806,-0.335467183812974,2.59501419582854));
#8466=CARTESIAN_POINT('Ctrl Pts',(7.19838636703693,-0.444497554803198,2.64699296075227));
#8467=CARTESIAN_POINT('Ctrl Pts',(7.51396784981042,-0.313675439428632,2.70919005501935));
#8468=CARTESIAN_POINT('Ctrl Pts',(7.62212313812957,-0.0514208051434247,
2.76101600110827));
#8469=CARTESIAN_POINT('Ctrl Pts',(7.57941022831611,0.159498854704775,2.80255943176652));
#8470=CARTESIAN_POINT('Ctrl Pts',(7.49002790476542,0.293811387305209,2.83377939972915));
#8471=CARTESIAN_POINT('Ctrl Pts',(7.3552499441484,0.383795703607156,2.86508254302445));
#8472=CARTESIAN_POINT('Ctrl Pts',(7.19595280633545,0.41560735445773,2.89648910888395));
#8473=CARTESIAN_POINT('Ctrl Pts',(7.03593949389396,0.383792650446306,2.92801879141503));
#8474=CARTESIAN_POINT('Ctrl Pts',(6.89961651509014,0.292876470296345,2.95969053299985));
#8475=CARTESIAN_POINT('Ctrl Pts',(6.8081238548802,0.155952445855146,2.99152250722056));
#8476=CARTESIAN_POINT('Ctrl Pts',(6.7719951154116,-0.0244720795860329,3.02708849903104));
#8477=CARTESIAN_POINT('Ctrl Pts',(6.82508694038131,-0.224423780156864,3.0664872528009));
#8478=CARTESIAN_POINT('Ctrl Pts',(6.9861130399098,-0.385566648672682,3.1098474493302));
#8479=CARTESIAN_POINT('Ctrl Pts',(7.18949761386412,-0.440411898981026,3.14997109794484));
#8480=CARTESIAN_POINT('Ctrl Pts',(7.37626527013998,-0.403213775048244,3.18676673081186));
#8481=CARTESIAN_POINT('Ctrl Pts',(7.51993103796524,-0.30750405465344,3.2201390303787));
#8482=CARTESIAN_POINT('Ctrl Pts',(7.61665044076158,-0.16281791922389,3.25377599756719));
#8483=CARTESIAN_POINT('Ctrl Pts',(7.65498225700094,0.0283123086785322,3.29145196922942));
#8484=CARTESIAN_POINT('Ctrl Pts',(7.59852316170633,0.240631420079613,3.3332902111484));
#8485=CARTESIAN_POINT('Ctrl Pts',(7.42736589163809,0.412328652603764,3.37943210760514));
#8486=CARTESIAN_POINT('Ctrl Pts',(7.19081184831391,0.475941162716025,3.42607713455886));
#8487=CARTESIAN_POINT('Ctrl Pts',(6.95151342469985,0.412204069493947,3.47322302929114));
#8488=CARTESIAN_POINT('Ctrl Pts',(6.77437422620912,0.235528496642651,3.52086247665056));
#8489=CARTESIAN_POINT('Ctrl Pts',(6.70856719057301,-0.00853695568196444,
3.56898306053165));
#8490=CARTESIAN_POINT('Ctrl Pts',(6.77444746404088,-0.255049338492359,3.61756749823055));
#8491=CARTESIAN_POINT('Ctrl Pts',(6.9562898685306,-0.437346140614658,3.66659366870206));
#8492=CARTESIAN_POINT('Ctrl Pts',(7.20705837195632,-0.504822359013845,3.71603499825878));
#8493=CARTESIAN_POINT('Ctrl Pts',(7.45987118758895,-0.437340247483335,3.76586064283255));
#8494=CARTESIAN_POINT('Ctrl Pts',(7.64643847266503,-0.251145802482984,3.81603581337119));
#8495=CARTESIAN_POINT('Ctrl Pts',(7.70939130979041,-0.0164226811455054,
3.86231497498143));
#8496=CARTESIAN_POINT('Ctrl Pts',(7.66665300702434,0.198091300428752,3.90458351454994));
#8497=CARTESIAN_POINT('Ctrl Pts',(7.55703831361006,0.362363180751678,3.94275824199772));
#8498=CARTESIAN_POINT('Ctrl Pts',(7.39231161872226,0.472405147713809,3.98104671473859));
#8499=CARTESIAN_POINT('Ctrl Pts',(7.19757748614764,0.511253819560404,4.01942894411337));
#8500=CARTESIAN_POINT('Ctrl Pts',(7.00243742159468,0.472394913482402,4.05788442705078));
#8501=CARTESIAN_POINT('Ctrl Pts',(6.83675859423202,0.361776141956741,4.09639221672569));
#8502=CARTESIAN_POINT('Ctrl Pts',(6.72593678453896,0.195994806221917,4.13493108529455));
#8503=CARTESIAN_POINT('Ctrl Pts',(6.6870196897812,0.000372767277272366,
4.17347960299015));
#8504=CARTESIAN_POINT('Ctrl Pts',(6.72599808190112,-0.19515902350661,4.21201632288769));
#8505=CARTESIAN_POINT('Ctrl Pts',(6.83662574734572,-0.360840864201945,4.25051978478148));
#8506=CARTESIAN_POINT('Ctrl Pts',(7.00208504736442,-0.47127212461887,4.28896891774833));
#8507=CARTESIAN_POINT('Ctrl Pts',(7.19679737636779,-0.510060779189973,4.32734248506513));
#8508=CARTESIAN_POINT('Ctrl Pts',(7.39100313831524,-0.471299286801184,4.36562087591661));
#8509=CARTESIAN_POINT('Ctrl Pts',(7.5551719819179,-0.361667391724164,4.40378216412631));
#8510=CARTESIAN_POINT('Ctrl Pts',(7.66435033350436,-0.197951056928272,4.44181269280615));
#8511=CARTESIAN_POINT('Ctrl Pts',(7.68982126235038,-0.0699660743691742,
4.46705762798012));
#8512=CARTESIAN_POINT('Ctrl Pts',(7.68982990724746,-0.00583191542195246,
4.4796574990714));
#8513=CARTESIAN_POINT('Origin',(7.65,-6.66133814775094E-16,4.45));
#8514=CARTESIAN_POINT('Origin',(7.65,-6.66133814775094E-16,4.45));
#8515=CARTESIAN_POINT('Origin',(7.65,-1.95245324213388E-18,0.55));
#9967=UNCERTAINTY_MEASURE_WITH_UNIT(LENGTH_MEASURE(0.001),#10021,
'DISTANCE_ACCURACY_VALUE',
'Maximum model space distance between geometric entities at asserted c
onnectivities');
#9987=UNCERTAINTY_MEASURE_WITH_UNIT(LENGTH_MEASURE(0.001),#10021,
'DISTANCE_ACCURACY_VALUE',
'Maximum model space distance between geometric entities at asserted c
onnectivities');
#10000=(
GEOMETRIC_REPRESENTATION_CONTEXT(3)
GLOBAL_UNCERTAINTY_ASSIGNED_CONTEXT((#9967))
GLOBAL_UNIT_ASSIGNED_CONTEXT((#10021,#10023,#10024))
REPRESENTATION_CONTEXT('','3D')
);
#10020=(
GEOMETRIC_REPRESENTATION_CONTEXT(3)
GLOBAL_UNCERTAINTY_ASSIGNED_CONTEXT((#9987))
GLOBAL_UNIT_ASSIGNED_CONTEXT((#10021,#10023,#10024))
REPRESENTATION_CONTEXT('','3D')
);
#10021=(
LENGTH_UNIT()
NAMED_UNIT(*)
SI_UNIT(.CENTI.,.METRE.)
);
#10023=(
NAMED_UNIT(*)
PLANE_ANGLE_UNIT()
SI_UNIT($,.RADIAN.)
);
#10024=(
NAMED_UNIT(*)
SI_UNIT($,.STERADIAN.)
SOLID_ANGLE_UNIT()
);
#10037=SHAPE_DEFINITION_REPRESENTATION(#10069,#10147);
#10069=PRODUCT_DEFINITION_SHAPE('',$,#10180);
#10147=SHAPE_REPRESENTATION('',(#5046),#10000);
#10167=PRODUCT_DEFINITION_CONTEXT('part definition',#10265,'design');
#10180=PRODUCT_DEFINITION('Installed compression spring',
'Installed compression spring',#10212,#10167);
#10212=PRODUCT_DEFINITION_FORMATION('',$,#10279);
#10265=APPLICATION_CONTEXT(
'Core Data for Automotive Mechanical Design Process');
#10266=PRODUCT_CONTEXT('part definition',#10265,'mechanical');
#10279=PRODUCT('Installed compression spring',
'Installed compression spring','Installed compression spring',(#10266));
#10362=COLOUR_RGB('Grey',0.48,0.52,0.57);
#10363=FILL_AREA_STYLE_COLOUR('',#10362);
#10364=FILL_AREA_STYLE('',(#10363));
#10365=SURFACE_STYLE_FILL_AREA(#10364);
#10366=SURFACE_SIDE_STYLE('',(#10365));
#10367=SURFACE_STYLE_USAGE(.BOTH.,#10366);
#10368=PRESENTATION_STYLE_ASSIGNMENT((#10367));
ENDSEC;
END-ISO-10303-21;
